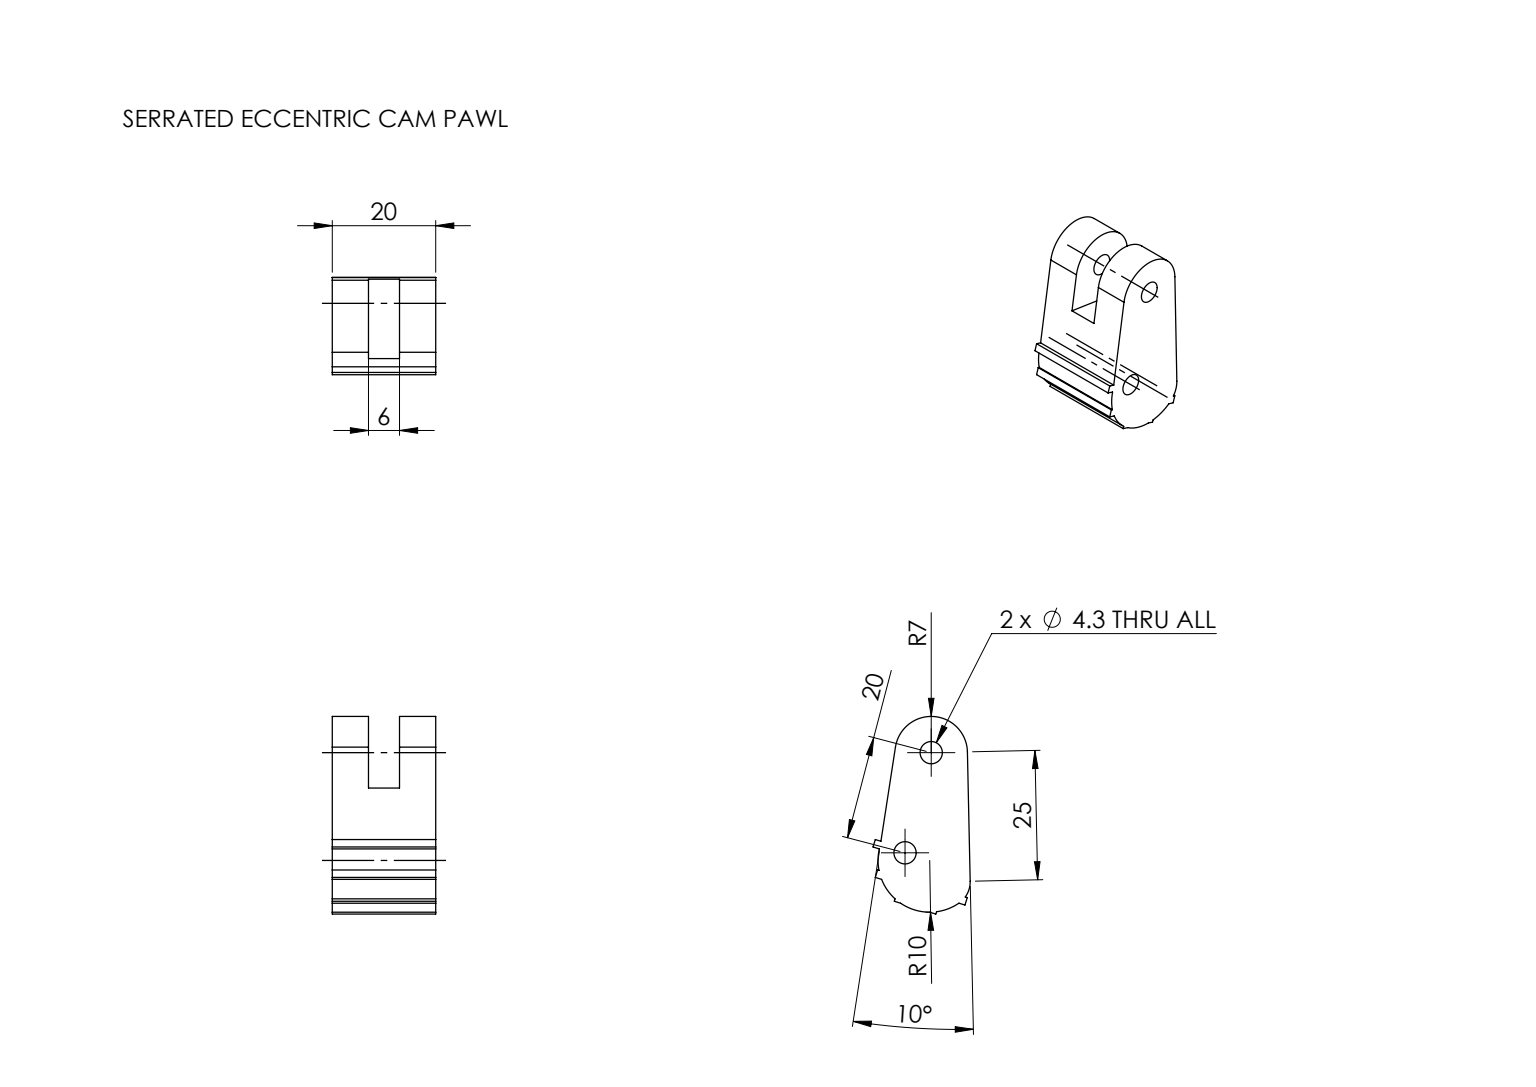
ISO-10303-21;
HEADER;
FILE_DESCRIPTION (('STEP AP214'),
    '1' );
FILE_NAME ('Serrated Eccentric Cam Pawl.step',
    '2026-10-03T20:08:58',
    ( '' ),
    ( '' ),
    'SwSTEP 2.0',
    'SolidWorks 2026',
    '' );
FILE_SCHEMA (( 'AUTOMOTIVE_DESIGN' ));
ENDSEC;

DATA;
#15=PLANE ( 'NONE',  #8371 ) ;
#32=AXIS2_PLACEMENT_3D ( 'NONE', #10637, #3883, #7557 ) ;
#37=ORIENTED_EDGE ( 'NONE', *, *, #5489, .T. ) ;
#60=VECTOR ( 'NONE', #10370, 1000.000000000000000 ) ;
#62=EDGE_CURVE ( 'NONE', #1807, #9471, #2410, .T. ) ;
#89=EDGE_CURVE ( 'NONE', #11132, #9471, #8961, .T. ) ;
#95=CARTESIAN_POINT ( 'NONE',  ( 20.00000000000000000, 39.49790820824818383, -24.06186359251417883 ) ) ;
#99=SHAPE_DEFINITION_REPRESENTATION ( #6268, #1377 ) ;
#101=ORIENTED_EDGE ( 'NONE', *, *, #1479, .F. ) ;
#103=ORIENTED_EDGE ( 'NONE', *, *, #2776, .T. ) ;
#110=ORIENTED_EDGE ( 'NONE', *, *, #895, .F. ) ;
#112=EDGE_CURVE ( 'NONE', #3836, #11042, #11228, .T. ) ;
#118=DIRECTION ( 'NONE',  ( 1.238279320584846685E-16, -0.9554649393887558739, 0.2951046417778634412 ) ) ;
#121=FACE_OUTER_BOUND ( 'NONE', #12151, .T. ) ;
#127=ORIENTED_EDGE ( 'NONE', *, *, #89, .F. ) ;
#135=CARTESIAN_POINT ( 'NONE',  ( 40.00000000000000711, 9.597108420813798446, -18.39576936187866352 ) ) ;
#149=CARTESIAN_POINT ( 'NONE',  ( 20.00000000000000355, 19.99999999999999645, -9.850000000000008527 ) ) ;
#155=ORIENTED_EDGE ( 'NONE', *, *, #11867, .F. ) ;
#170=CARTESIAN_POINT ( 'NONE',  ( 20.00000000000000355, 10.25912655421750230, -11.14847175327133577 ) ) ;
#172=ORIENTED_EDGE ( 'NONE', *, *, #1630, .T. ) ;
#199=AXIS2_PLACEMENT_3D ( 'NONE', #4415, #11118, #3403 ) ;
#205=AXIS2_PLACEMENT_3D ( 'NONE', #5168, #9083, #12128 ) ;
#211=CARTESIAN_POINT ( 'NONE',  ( 27.00000000000000355, 39.34792583643766051, -14.91347054209568945 ) ) ;
#216=CARTESIAN_POINT ( 'NONE',  ( 40.00000000000000000, 39.34792583643765340, -17.06347054209567560 ) ) ;
#220=ADVANCED_FACE ( 'NONE', ( #2602 ), #12455, .T. ) ;
#231=CARTESIAN_POINT ( 'NONE',  ( 40.00000000000000711, 10.63631887905126128, -9.927230231572499619 ) ) ;
#238=ORIENTED_EDGE ( 'NONE', *, *, #6687, .T. ) ;
#243=ORIENTED_EDGE ( 'NONE', *, *, #11135, .T. ) ;
#264=AXIS2_PLACEMENT_3D ( 'NONE', #2269, #10097, #5222 ) ;
#268=EDGE_CURVE ( 'NONE', #6675, #6031, #2672, .T. ) ;
#277=DIRECTION ( 'NONE',  ( -0.000000000000000000, -0.9883022714608525883, 0.1525077710325583313 ) ) ;
#304=EDGE_CURVE ( 'NONE', #11281, #1954, #7365, .T. ) ;
#316=ORIENTED_EDGE ( 'NONE', *, *, #9501, .T. ) ;
#357=LINE ( 'NONE', #2369, #4310 ) ;
#367=ADVANCED_FACE ( 'NONE', ( #4841 ), #6716, .F. ) ;
#385=LINE ( 'NONE', #10217, #5971 ) ;
#407=DIRECTION ( 'NONE',  ( 0.000000000000000000, 1.000000000000000000, 0.000000000000000000 ) ) ;
#416=VECTOR ( 'NONE', #1989, 1000.000000000000114 ) ;
#421=CARTESIAN_POINT ( 'NONE',  ( 40.00000000000000711, 18.52447679111068268, -16.77732469694377926 ) ) ;
#424=ORIENTED_EDGE ( 'NONE', *, *, #89, .T. ) ;
#425=DIRECTION ( 'NONE',  ( 0.000000000000000000, -0.9554649393887557629, 0.2951046417778634412 ) ) ;
#427=ORIENTED_EDGE ( 'NONE', *, *, #12083, .T. ) ;
#430=ORIENTED_EDGE ( 'NONE', *, *, #2792, .F. ) ;
#431=DIRECTION ( 'NONE',  ( 0.000000000000000000, -0.2951046417778627751, -0.9554649393887560960 ) ) ;
#433=SURFACE_SIDE_STYLE ('',( #11389 ) ) ;
#460=VECTOR ( 'NONE', #2524, 1000.000000000000000 ) ;
#463=EDGE_LOOP ( 'NONE', ( #110, #9977 ) ) ;
#484=CYLINDRICAL_SURFACE ( 'NONE', #199, 10.00000000000000000 ) ;
#488=AXIS2_PLACEMENT_3D ( 'NONE', #8589, #5753, #5691 ) ;
#489=FACE_BOUND ( 'NONE', #6630, .T. ) ;
#496=PLANE ( 'NONE',  #10808 ) ;
#500=DIRECTION ( 'NONE',  ( 0.000000000000000000, -0.9554649393887557629, 0.2951046417778634412 ) ) ;
#505=CARTESIAN_POINT ( 'NONE',  ( 20.00000000000000000, 21.12780530657007461, -5.807015647486883481 ) ) ;
#511=CARTESIAN_POINT ( 'NONE',  ( 40.00000000000000711, 15.24625277455639250, -6.248133273622505257 ) ) ;
#553=VECTOR ( 'NONE', #2820, 1000.000000000000114 ) ;
#557=ORIENTED_EDGE ( 'NONE', *, *, #3842, .T. ) ;
#563=VECTOR ( 'NONE', #1495, 1000.000000000000227 ) ;
#567=CARTESIAN_POINT ( 'NONE',  ( 40.00000000000000000, 39.49790820824818383, -24.06186359251417883 ) ) ;
#570=CARTESIAN_POINT ( 'NONE',  ( 40.00000000000000711, 19.99999999999999645, -14.14999999999999147 ) ) ;
#574=VERTEX_POINT ( 'NONE', #5990 ) ;
#575=DIRECTION ( 'NONE',  ( 1.238279320584846685E-16, -0.9554649393887560960, 0.2951046417778627751 ) ) ;
#577=DIRECTION ( 'NONE',  ( -1.000000000000000000, -1.081682119347366197E-16, 6.938893903907228378E-17 ) ) ;
#578=EDGE_CURVE ( 'NONE', #7319, #12298, #9904, .T. ) ;
#580=CYLINDRICAL_SURFACE ( 'NONE', #12033, 2.149999999999992362 ) ;
#614=CARTESIAN_POINT ( 'NONE',  ( 20.00000000000000000, 11.34118543499637077, -24.03007857557328464 ) ) ;
#615=ADVANCED_FACE ( 'NONE', ( #7162 ), #11080, .F. ) ;
#616=CARTESIAN_POINT ( 'NONE',  ( 20.00000000000000355, 18.52447679111067913, -16.77732469694377926 ) ) ;
#621=CIRCLE ( 'NONE', #7816, 9.999999999999998224 ) ;
#642=CARTESIAN_POINT ( 'NONE',  ( 33.00000000000000000, 14.50364731389636397, -24.59751492040896892 ) ) ;
#643=DIRECTION ( 'NONE',  ( 0.000000000000000000, 0.000000000000000000, -1.000000000000000000 ) ) ;
#665=ORIENTED_EDGE ( 'NONE', *, *, #1472, .F. ) ;
#671=CIRCLE ( 'NONE', #10117, 2.149999999999985256 ) ;
#695=EDGE_CURVE ( 'NONE', #11780, #5322, #2587, .T. ) ;
#699=DIRECTION ( 'NONE',  ( 1.000000000000000000, 1.081682119347366197E-16, -6.938893903907228378E-17 ) ) ;
#702=CARTESIAN_POINT ( 'NONE',  ( 27.00000000000000355, 29.58047730022061472, -27.90351864933187898 ) ) ;
#713=CARTESIAN_POINT ( 'NONE',  ( 40.00000000000000711, 11.34118543499637255, -24.03007857557328464 ) ) ;
#725=CARTESIAN_POINT ( 'NONE',  ( 20.00000000000000000, 12.07894703944102766, -21.64141622710139146 ) ) ;
#728=ORIENTED_EDGE ( 'NONE', *, *, #9809, .F. ) ;
#733=LINE ( 'NONE', #12601, #6869 ) ;
#762=CARTESIAN_POINT ( 'NONE',  ( 40.00000000000000711, 10.26855730552414059, -22.42000078613342851 ) ) ;
#767=CARTESIAN_POINT ( 'NONE',  ( 40.00000000000000711, 30.14235464176399404, -24.26236220746664785 ) ) ;
#779=CARTESIAN_POINT ( 'NONE',  ( 20.00000000000000000, 10.63631887905125950, -9.927230231572497843 ) ) ;
#805=CARTESIAN_POINT ( 'NONE',  ( 40.00000000000000711, 11.45997319858344987, -23.64547756539572276 ) ) ;
#821=AXIS2_PLACEMENT_3D ( 'NONE', #5989, #11671, #5736 ) ;
#824=EDGE_CURVE ( 'NONE', #7005, #11281, #3866, .T. ) ;
#850=DIRECTION ( 'NONE',  ( 1.000000000000000000, -0.000000000000000000, -6.938893903907228378E-17 ) ) ;
#862=ORIENTED_EDGE ( 'NONE', *, *, #6687, .F. ) ;
#872=EDGE_CURVE ( 'NONE', #5322, #574, #6832, .T. ) ;
#876=LINE ( 'NONE', #4088, #7398 ) ;
#879=EDGE_LOOP ( 'NONE', ( #430, #5834, #11812, #1139 ) ) ;
#895=EDGE_CURVE ( 'NONE', #6619, #5731, #4929, .T. ) ;
#913=VECTOR ( 'NONE', #8680, 1000.000000000000000 ) ;
#915=DIRECTION ( 'NONE',  ( -1.000000000000000000, -1.081682119347366197E-16, 6.938893903907228378E-17 ) ) ;
#923=CARTESIAN_POINT ( 'NONE',  ( 20.00000000000000000, 8.163911011730665024, -17.95311239921186441 ) ) ;
#925=EDGE_CURVE ( 'NONE', #10658, #2655, #357, .T. ) ;
#938=VERTEX_POINT ( 'NONE', #7194 ) ;
#946=DIRECTION ( 'NONE',  ( -1.081682119347366197E-16, 1.000000000000000000, 0.000000000000000000 ) ) ;
#948=ADVANCED_FACE ( 'NONE', ( #3466 ), #484, .T. ) ;
#950=ORIENTED_EDGE ( 'NONE', *, *, #1873, .F. ) ;
#964=EDGE_CURVE ( 'NONE', #11709, #1279, #2236, .T. ) ;
#970=DIRECTION ( 'NONE',  ( 7.169062767534772867E-17, -0.02142605311579142552, 0.9997704357740727632 ) ) ;
#997=EDGE_CURVE ( 'NONE', #3286, #9151, #3483, .T. ) ;
#1008=EDGE_LOOP ( 'NONE', ( #5764, #10223, #12292, #11299 ) ) ;
#1031=CARTESIAN_POINT ( 'NONE',  ( 40.00000000000000711, 14.50364731389636574, -24.59751492040896892 ) ) ;
#1037=CYLINDRICAL_SURFACE ( 'NONE', #1434, 10.00000000000000000 ) ;
#1101=DIRECTION ( 'NONE',  ( 1.238279320584846685E-16, -0.9554649393887560960, 0.2951046417778627751 ) ) ;
#1122=ORIENTED_EDGE ( 'NONE', *, *, #9718, .T. ) ;
#1131=CARTESIAN_POINT ( 'NONE',  ( 20.00000000000000355, 19.99999999999999645, -12.00000000000000000 ) ) ;
#1138=VECTOR ( 'NONE', #1770, 1000.000000000000000 ) ;
#1139=ORIENTED_EDGE ( 'NONE', *, *, #8439, .F. ) ;
#1152=CARTESIAN_POINT ( 'NONE',  ( 40.00000000000000711, 8.524476791110680907, -16.77732469694377926 ) ) ;
#1163=CARTESIAN_POINT ( 'NONE',  ( 20.00000000000000000, 15.24625277455639072, -6.248133273622503481 ) ) ;
#1190=DIRECTION ( 'NONE',  ( 1.000000000000000000, -0.000000000000000000, -6.938893903907228378E-17 ) ) ;
#1192=DIRECTION ( 'NONE',  ( 1.000000000000000000, 1.081682119347366197E-16, -6.938893903907228378E-17 ) ) ;
#1195=EDGE_CURVE ( 'NONE', #8729, #11132, #8527, .T. ) ;
#1202=DIRECTION ( 'NONE',  ( 0.000000000000000000, 1.000000000000000000, 0.000000000000000000 ) ) ;
#1205=CIRCLE ( 'NONE', #11288, 9.999999999999998224 ) ;
#1212=CIRCLE ( 'NONE', #9019, 2.149999999999985256 ) ;
#1235=EDGE_LOOP ( 'NONE', ( #8347, #1122, #10045, #7560 ) ) ;
#1245=EDGE_CURVE ( 'NONE', #6857, #5859, #1205, .T. ) ;
#1251=CARTESIAN_POINT ( 'NONE',  ( 40.00000000000000000, 39.34792583643766051, -14.91347054209569301 ) ) ;
#1254=ORIENTED_EDGE ( 'NONE', *, *, #1536, .F. ) ;
#1258=DIRECTION ( 'NONE',  ( 1.000000000000000000, 1.081682119347366321E-16, -6.938893903907228378E-17 ) ) ;
#1279=VERTEX_POINT ( 'NONE', #1952 ) ;
#1322=CARTESIAN_POINT ( 'NONE',  ( 40.00000000000000000, 39.34792583643766051, -19.21347054209566352 ) ) ;
#1323=DIRECTION ( 'NONE',  ( -3.437775699846489820E-17, -0.2951046417778627751, -0.9554649393887560960 ) ) ;
#1333=LINE ( 'NONE', #5084, #4298 ) ;
#1340=CYLINDRICAL_SURFACE ( 'NONE', #12047, 10.00000000000000000 ) ;
#1348=CARTESIAN_POINT ( 'NONE',  ( 40.00000000000000711, 10.63631887905126128, -9.927230231572499619 ) ) ;
#1377=SHAPE_REPRESENTATION ( 'Serrated Eccentric Cam Pawl', ( #12422 ), #2062 ) ;
#1394=EDGE_CURVE ( 'NONE', #8136, #2021, #2508, .T. ) ;
#1410=DIRECTION ( 'NONE',  ( 1.000000000000000000, 1.081682119347366321E-16, -6.938893903907228378E-17 ) ) ;
#1427=VERTEX_POINT ( 'NONE', #7520 ) ;
#1434=AXIS2_PLACEMENT_3D ( 'NONE', #9786, #915, #4065 ) ;
#1438=ORIENTED_EDGE ( 'NONE', *, *, #11480, .F. ) ;
#1442=MECHANICAL_DESIGN_GEOMETRIC_PRESENTATION_REPRESENTATION('',(#12570),#6396);
#1462=LINE ( 'NONE', #3417, #2826 ) ;
#1472=EDGE_CURVE ( 'NONE', #11132, #938, #6627, .T. ) ;
#1479=EDGE_CURVE ( 'NONE', #6979, #2021, #10668, .T. ) ;
#1495=DIRECTION ( 'NONE',  ( 2.187388225841179596E-16, -0.9997704357740726522, -0.02142605311579142552 ) ) ;
#1499=CARTESIAN_POINT ( 'NONE',  ( 20.00000000000000000, 21.12780530657007461, -5.807015647486883481 ) ) ;
#1517=EDGE_LOOP ( 'NONE', ( #10586, #238, #7027, #9677, #2521, #5666, #4792, #7574 ) ) ;
#1536=EDGE_CURVE ( 'NONE', #4933, #5862, #5134, .T. ) ;
#1546=VECTOR ( 'NONE', #10772, 1000.000000000000000 ) ;
#1555=DIRECTION ( 'NONE',  ( 1.000000000000000000, 1.081682119347366197E-16, -6.938893903907228378E-17 ) ) ;
#1560=CARTESIAN_POINT ( 'NONE',  ( 20.00000000000000355, 8.611173066148735344, -18.09125363591105540 ) ) ;
#1563=CYLINDRICAL_SURFACE ( 'NONE', #12684, 5.000000000000000888 ) ;
#1589=DIRECTION ( 'NONE',  ( -1.081682119347366197E-16, 1.000000000000000000, 0.000000000000000000 ) ) ;
#1597=VECTOR ( 'NONE', #10603, 1000.000000000000000 ) ;
#1599=CARTESIAN_POINT ( 'NONE',  ( 40.00000000000000711, 22.22477142302764364, -7.338293953734280173 ) ) ;
#1630=EDGE_CURVE ( 'NONE', #6277, #6857, #876, .T. ) ;
#1651=AXIS2_PLACEMENT_3D ( 'NONE', #11186, #8281, #2434 ) ;
#1656=DIRECTION ( 'NONE',  ( 1.000000000000000000, 1.081682119347366197E-16, -6.938893903907228378E-17 ) ) ;
#1698=EDGE_LOOP ( 'NONE', ( #12167, #10076, #4423, #3828 ) ) ;
#1714=ORIENTED_EDGE ( 'NONE', *, *, #8066, .F. ) ;
#1715=ORIENTED_EDGE ( 'NONE', *, *, #3433, .F. ) ;
#1735=CARTESIAN_POINT ( 'NONE',  ( 40.00000000000000711, 12.07894703944102943, -21.64141622710139146 ) ) ;
#1737=DIRECTION ( 'NONE',  ( 0.000000000000000000, 0.000000000000000000, -1.000000000000000000 ) ) ;
#1770=DIRECTION ( 'NONE',  ( 1.238279320584846685E-16, -0.9554649393887558739, 0.2951046417778634412 ) ) ;
#1772=STYLED_ITEM ( 'NONE', ( #12365 ), #5705 ) ;
#1776=CARTESIAN_POINT ( 'NONE',  ( 20.00000000000000000, 10.63631887905125950, -9.927230231572497843 ) ) ;
#1799=CARTESIAN_POINT ( 'NONE',  ( 20.00000000000000000, 10.64574963035789601, -21.19875926443459591 ) ) ;
#1807=VERTEX_POINT ( 'NONE', #12615 ) ;
#1819=FACE_OUTER_BOUND ( 'NONE', #3970, .T. ) ;
#1822=VERTEX_POINT ( 'NONE', #10654 ) ;
#1839=EDGE_CURVE ( 'NONE', #5204, #2655, #5643, .T. ) ;
#1869=CARTESIAN_POINT ( 'NONE',  ( 40.00000000000000711, 14.86906044972264240, -7.469374795321334304 ) ) ;
#1873=EDGE_CURVE ( 'NONE', #9471, #9760, #10978, .T. ) ;
#1899=ORIENTED_EDGE ( 'NONE', *, *, #578, .T. ) ;
#1915=ORIENTED_EDGE ( 'NONE', *, *, #2093, .T. ) ;
#1952=CARTESIAN_POINT ( 'NONE',  ( 40.00000000000000711, 10.25912655421750230, -11.14847175327134110 ) ) ;
#1954=VERTEX_POINT ( 'NONE', #11894 ) ;
#1984=CIRCLE ( 'NONE', #6311, 2.149999999999985256 ) ;
#1986=CARTESIAN_POINT ( 'NONE',  ( 32.99999999999999289, 39.34792583643766051, -14.91347054209568945 ) ) ;
#1989=DIRECTION ( 'NONE',  ( -0.000000000000000000, -0.9883022714608525883, 0.1525077710325583313 ) ) ;
#1993=EDGE_LOOP ( 'NONE', ( #10669, #10613, #8744, #5830 ) ) ;
#2003=DIRECTION ( 'NONE',  ( -3.437775699846489820E-17, -0.2951046417778627751, -0.9554649393887560960 ) ) ;
#2004=PLANE ( 'NONE',  #7497 ) ;
#2021=VERTEX_POINT ( 'NONE', #1251 ) ;
#2023=ORIENTED_EDGE ( 'NONE', *, *, #11135, .F. ) ;
#2026=DIRECTION ( 'NONE',  ( -3.437775699846489820E-17, -0.2951046417778627751, -0.9554649393887560960 ) ) ;
#2047=VECTOR ( 'NONE', #3153, 1000.000000000000114 ) ;
#2049=CARTESIAN_POINT ( 'NONE',  ( 20.00000000000000000, 11.10553687445042570, -10.07215277424222855 ) ) ;
#2062=( GEOMETRIC_REPRESENTATION_CONTEXT ( 3 ) GLOBAL_UNCERTAINTY_ASSIGNED_CONTEXT ( ( #5469 ) ) GLOBAL_UNIT_ASSIGNED_CONTEXT ( ( #2406, #6390, #11551 ) ) REPRESENTATION_CONTEXT ( 'NONE', 'WORKASPACE' ) );
#2075=CARTESIAN_POINT ( 'NONE',  ( 20.00000000000000000, 15.24625277455639072, -6.248133273622503481 ) ) ;
#2093=EDGE_CURVE ( 'NONE', #6823, #9939, #4104, .T. ) ;
#2103=LINE ( 'NONE', #4160, #8896 ) ;
#2127=VERTEX_POINT ( 'NONE', #6657 ) ;
#2147=EDGE_CURVE ( 'NONE', #12369, #1954, #4712, .T. ) ;
#2148=DIRECTION ( 'NONE',  ( -1.000000000000000000, -2.206481006425900381E-16, 8.674603474570137221E-17 ) ) ;
#2153=EDGE_LOOP ( 'NONE', ( #101, #3167 ) ) ;
#2165=CARTESIAN_POINT ( 'NONE',  ( 40.00000000000000711, 22.56100271565320980, -6.249672610153679919 ) ) ;
#2181=CARTESIAN_POINT ( 'NONE',  ( 27.00000000000000355, 39.34792583643766051, -17.06347054209567915 ) ) ;
#2190=FACE_OUTER_BOUND ( 'NONE', #11323, .T. ) ;
#2193=ADVANCED_FACE ( 'NONE', ( #3115 ), #11861, .T. ) ;
#2206=ADVANCED_BREP_SHAPE_REPRESENTATION ( '', ( #5705, #12422 ), #2062 ) ;
#2209=CARTESIAN_POINT ( 'NONE',  ( 32.99999999999999289, 39.34792583643766051, -19.21347054209566707 ) ) ;
#2225=DIRECTION ( 'NONE',  ( 0.000000000000000000, -1.000000000000000000, 0.000000000000000000 ) ) ;
#2226=ORIENTED_EDGE ( 'NONE', *, *, #7584, .T. ) ;
#2232=EDGE_LOOP ( 'NONE', ( #3487, #155, #2650, #1915 ) ) ;
#2236=LINE ( 'NONE', #231, #4108 ) ;
#2246=CARTESIAN_POINT ( 'NONE',  ( 40.00000000000000711, 14.86906044972263707, -7.469374795321336080 ) ) ;
#2269=CARTESIAN_POINT ( 'NONE',  ( 40.00000000000000000, 39.34792583643766051, -17.06347054209567915 ) ) ;
#2289=DIRECTION ( 'NONE',  ( -1.000000000000000000, -1.081682119347366197E-16, 6.938893903907228378E-17 ) ) ;
#2308=ORIENTED_EDGE ( 'NONE', *, *, #9718, .F. ) ;
#2323=FACE_OUTER_BOUND ( 'NONE', #2841, .T. ) ;
#2329=DIRECTION ( 'NONE',  ( -3.437775699846489820E-17, -0.2951046417778627751, -0.9554649393887560960 ) ) ;
#2369=CARTESIAN_POINT ( 'NONE',  ( 20.00000000000000000, 10.63631887905125950, -9.927230231572497843 ) ) ;
#2370=FACE_OUTER_BOUND ( 'NONE', #9107, .T. ) ;
#2373=PLANE ( 'NONE',  #10491 ) ;
#2401=FACE_OUTER_BOUND ( 'NONE', #9363, .T. ) ;
#2406=( LENGTH_UNIT ( ) NAMED_UNIT ( * ) SI_UNIT ( .MILLI., .METRE. ) );
#2410=LINE ( 'NONE', #11095, #4379 ) ;
#2420=FACE_OUTER_BOUND ( 'NONE', #6608, .T. ) ;
#2428=CARTESIAN_POINT ( 'NONE',  ( 20.00000000000000355, 19.99999999999999645, -12.00000000000000000 ) ) ;
#2432=EDGE_CURVE ( 'NONE', #8348, #4291, #385, .T. ) ;
#2434=DIRECTION ( 'NONE',  ( 0.000000000000000000, -1.000000000000000000, 0.000000000000000000 ) ) ;
#2439=EDGE_CURVE ( 'NONE', #8682, #11780, #6642, .T. ) ;
#2451=VERTEX_POINT ( 'NONE', #4642 ) ;
#2480=EDGE_CURVE ( 'NONE', #3728, #7005, #3105, .T. ) ;
#2483=CARTESIAN_POINT ( 'NONE',  ( 40.00000000000000000, 39.49790820824818383, -24.06186359251417883 ) ) ;
#2504=ORIENTED_EDGE ( 'NONE', *, *, #6586, .T. ) ;
#2506=FACE_BOUND ( 'NONE', #463, .T. ) ;
#2508=LINE ( 'NONE', #2712, #7385 ) ;
#2520=EDGE_CURVE ( 'NONE', #574, #12468, #4580, .T. ) ;
#2521=ORIENTED_EDGE ( 'NONE', *, *, #5672, .F. ) ;
#2524=DIRECTION ( 'NONE',  ( -1.238279320584846685E-16, 0.9554649393887558739, -0.2951046417778634412 ) ) ;
#2550=EDGE_CURVE ( 'NONE', #11042, #11825, #10490, .T. ) ;
#2554=CARTESIAN_POINT ( 'NONE',  ( 20.00000000000000000, 16.59466514679920124, -6.965300083364789785 ) ) ;
#2562=ORIENTED_EDGE ( 'NONE', *, *, #5672, .T. ) ;
#2587=LINE ( 'NONE', #642, #11771 ) ;
#2602=FACE_OUTER_BOUND ( 'NONE', #12626, .T. ) ;
#2603=COLOUR_RGB ( '', 0.31764706, 0.68627451, 0.89019608) ;
#2604=CARTESIAN_POINT ( 'NONE',  ( 20.00000000000000355, 11.45997319858344810, -23.64547756539571566 ) ) ;
#2610=VECTOR ( 'NONE', #10522, 1000.000000000000000 ) ;
#2624=EDGE_CURVE ( 'NONE', #8729, #1807, #5914, .T. ) ;
#2629=CARTESIAN_POINT ( 'NONE',  ( 40.00000000000000711, 21.12780530657007816, -5.807015647486885257 ) ) ;
#2637=EDGE_CURVE ( 'NONE', #2127, #6031, #2789, .T. ) ;
#2644=EDGE_CURVE ( 'NONE', #1822, #11190, #12694, .T. ) ;
#2650=ORIENTED_EDGE ( 'NONE', *, *, #7602, .T. ) ;
#2655=VERTEX_POINT ( 'NONE', #2049 ) ;
#2665=PRESENTATION_STYLE_ASSIGNMENT (( #9584 ) ) ;
#2671=VECTOR ( 'NONE', #10863, 1000.000000000000000 ) ;
#2672=LINE ( 'NONE', #6394, #4168 ) ;
#2673=CARTESIAN_POINT ( 'NONE',  ( 40.00000000000000711, 19.99999999999999645, -12.00000000000000178 ) ) ;
#2689=ORIENTED_EDGE ( 'NONE', *, *, #4520, .T. ) ;
#2700=ORIENTED_EDGE ( 'NONE', *, *, #7431, .T. ) ;
#2712=CARTESIAN_POINT ( 'NONE',  ( 40.00000000000000000, 39.34792583643766051, -14.91347054209568945 ) ) ;
#2727=ADVANCED_FACE ( 'NONE', ( #3355 ), #3168, .F. ) ;
#2732=ORIENTED_EDGE ( 'NONE', *, *, #3539, .F. ) ;
#2768=ORIENTED_EDGE ( 'NONE', *, *, #9825, .T. ) ;
#2769=DIRECTION ( 'NONE',  ( -3.437775699846481192E-17, -0.2951046417778634967, -0.9554649393887558739 ) ) ;
#2776=EDGE_CURVE ( 'NONE', #11825, #1954, #1333, .T. ) ;
#2789=LINE ( 'NONE', #4767, #2671 ) ;
#2792=EDGE_CURVE ( 'NONE', #10595, #4775, #12045, .T. ) ;
#2800=CARTESIAN_POINT ( 'NONE',  ( 40.00000000000000711, 10.64574963035789779, -21.19875926443459591 ) ) ;
#2804=VECTOR ( 'NONE', #12374, 1000.000000000000114 ) ;
#2807=AXIS2_PLACEMENT_3D ( 'NONE', #6219, #3406, #425 ) ;
#2820=DIRECTION ( 'NONE',  ( -3.437775699846489820E-17, -0.2951046417778627751, -0.9554649393887560960 ) ) ;
#2826=VECTOR ( 'NONE', #7333, 1000.000000000000000 ) ;
#2841=EDGE_LOOP ( 'NONE', ( #12665, #10276, #10719, #8806 ) ) ;
#2852=ORIENTED_EDGE ( 'NONE', *, *, #5325, .F. ) ;
#2854=ORIENTED_EDGE ( 'NONE', *, *, #10288, .F. ) ;
#2873=UNCERTAINTY_MEASURE_WITH_UNIT (LENGTH_MEASURE( 1.000000000000000082E-05 ), #11195, 'distance_accuracy_value', 'NONE');
#2898=DIRECTION ( 'NONE',  ( -1.000000000000000000, -1.081682119347366197E-16, 6.938893903907228378E-17 ) ) ;
#2899=ORIENTED_EDGE ( 'NONE', *, *, #6245, .T. ) ;
#2911=ORIENTED_EDGE ( 'NONE', *, *, #10731, .T. ) ;
#2919=EDGE_CURVE ( 'NONE', #6872, #11175, #6360, .T. ) ;
#2936=DIRECTION ( 'NONE',  ( -1.000000000000000000, -2.206481006425900381E-16, 8.674603474570138454E-17 ) ) ;
#2938=AXIS2_PLACEMENT_3D ( 'NONE', #1031, #970, #8643 ) ;
#2951=DIRECTION ( 'NONE',  ( 0.000000000000000000, -0.2951046417778627751, -0.9554649393887560960 ) ) ;
#2956=ORIENTED_EDGE ( 'NONE', *, *, #2432, .T. ) ;
#3016=ORIENTED_EDGE ( 'NONE', *, *, #925, .F. ) ;
#3024=DIRECTION ( 'NONE',  ( -1.000000000000000000, -1.081682119347366197E-16, 6.938893903907228378E-17 ) ) ;
#3028=CARTESIAN_POINT ( 'NONE',  ( 40.00000000000000711, 19.99999999999999645, -9.850000000000010303 ) ) ;
#3038=DIRECTION ( 'NONE',  ( 1.000000000000000000, 1.081682119347366321E-16, -6.938893903907228378E-17 ) ) ;
#3087=AXIS2_PLACEMENT_3D ( 'NONE', #11131, #4300, #8164 ) ;
#3088=CARTESIAN_POINT ( 'NONE',  ( 40.00000000000000000, 39.34792583643766051, -17.06347054209567915 ) ) ;
#3105=CIRCLE ( 'NONE', #4536, 9.999999999999998224 ) ;
#3115=FACE_OUTER_BOUND ( 'NONE', #879, .T. ) ;
#3139=DIRECTION ( 'NONE',  ( 1.238279320584846685E-16, -0.9554649393887560960, 0.2951046417778627751 ) ) ;
#3153=DIRECTION ( 'NONE',  ( -3.437775699846489820E-17, -0.2951046417778627751, -0.9554649393887560960 ) ) ;
#3162=ORIENTED_EDGE ( 'NONE', *, *, #1839, .T. ) ;
#3167=ORIENTED_EDGE ( 'NONE', *, *, #12083, .F. ) ;
#3168=PLANE ( 'NONE',  #3087 ) ;
#3195=FACE_BOUND ( 'NONE', #9629, .T. ) ;
#3203=EDGE_CURVE ( 'NONE', #9222, #6979, #2103, .T. ) ;
#3205=CARTESIAN_POINT ( 'NONE',  ( 40.00000000000000711, 14.39651704831740986, -19.59866274153860388 ) ) ;
#3209=ORIENTED_EDGE ( 'NONE', *, *, #2644, .T. ) ;
#3221=LINE ( 'NONE', #9941, #7769 ) ;
#3225=CIRCLE ( 'NONE', #10383, 2.149999999999988809 ) ;
#3241=CARTESIAN_POINT ( 'NONE',  ( 20.00000000000000000, 9.597108420813796670, -18.39576936187866352 ) ) ;
#3258=EDGE_CURVE ( 'NONE', #9939, #10595, #12628, .T. ) ;
#3272=ORIENTED_EDGE ( 'NONE', *, *, #62, .T. ) ;
#3286=VERTEX_POINT ( 'NONE', #9409 ) ;
#3288=LINE ( 'NONE', #9182, #11387 ) ;
#3297=CARTESIAN_POINT ( 'NONE',  ( 20.00000000000000355, 14.50364731389636397, -24.59751492040896892 ) ) ;
#3329=CARTESIAN_POINT ( 'NONE',  ( 40.00000000000000711, 21.47552320888931021, -7.222675303056226070 ) ) ;
#3344=CARTESIAN_POINT ( 'NONE',  ( 20.00000000000000000, 10.63631887905125950, -9.927230231572497843 ) ) ;
#3355=FACE_OUTER_BOUND ( 'NONE', #3473, .T. ) ;
#3403=DIRECTION ( 'NONE',  ( 0.000000000000000000, -1.000000000000000000, 0.000000000000000000 ) ) ;
#3406=DIRECTION ( 'NONE',  ( 3.437775699846481192E-17, 0.2951046417778634967, 0.9554649393887558739 ) ) ;
#3415=DIRECTION ( 'NONE',  ( -1.000000000000000000, -2.206481006425900381E-16, 8.674603474570138454E-17 ) ) ;
#3417=CARTESIAN_POINT ( 'NONE',  ( 40.00000000000000711, 22.22477142302764008, -7.338293953734282837 ) ) ;
#3433=EDGE_CURVE ( 'NONE', #5862, #6619, #733, .T. ) ;
#3436=VECTOR ( 'NONE', #4384, 1000.000000000000000 ) ;
#3441=CARTESIAN_POINT ( 'NONE',  ( 40.00000000000000711, 8.611173066148737121, -18.09125363591105540 ) ) ;
#3450=FACE_OUTER_BOUND ( 'NONE', #12688, .T. ) ;
#3454=DIRECTION ( 'NONE',  ( 1.238279320584846685E-16, -0.9554649393887560960, 0.2951046417778627751 ) ) ;
#3466=FACE_OUTER_BOUND ( 'NONE', #4679, .T. ) ;
#3473=EDGE_LOOP ( 'NONE', ( #6548, #2562, #665, #424 ) ) ;
#3481=FACE_OUTER_BOUND ( 'NONE', #1993, .T. ) ;
#3483=CIRCLE ( 'NONE', #6962, 2.149999999999985256 ) ;
#3485=DIRECTION ( 'NONE',  ( 0.000000000000000000, -1.000000000000000000, 0.000000000000000000 ) ) ;
#3487=ORIENTED_EDGE ( 'NONE', *, *, #12307, .F. ) ;
#3489=DIRECTION ( 'NONE',  ( 0.000000000000000000, 1.000000000000000000, 0.000000000000000000 ) ) ;
#3498=PLANE ( 'NONE',  #205 ) ;
#3500=VECTOR ( 'NONE', #11205, 1000.000000000000000 ) ;
#3539=EDGE_CURVE ( 'NONE', #11717, #12369, #12634, .T. ) ;
#3568=DIRECTION ( 'NONE',  ( -1.000000000000000000, -1.081682119347366197E-16, 6.938893903907228378E-17 ) ) ;
#3599=FILL_AREA_STYLE_COLOUR ( '', #2603 ) ;
#3600=ORIENTED_EDGE ( 'NONE', *, *, #12188, .T. ) ;
#3609=DIRECTION ( 'NONE',  ( -3.437775699846489820E-17, -0.2951046417778627751, -0.9554649393887560960 ) ) ;
#3614=CARTESIAN_POINT ( 'NONE',  ( 20.00000000000000000, 39.34792583643765340, -17.06347054209567560 ) ) ;
#3620=ADVANCED_FACE ( 'NONE', ( #3195, #11942 ), #4204, .T. ) ;
#3635=DIRECTION ( 'NONE',  ( -1.000000000000000000, -1.081682119347366197E-16, 6.938893903907228378E-17 ) ) ;
#3646=DIRECTION ( 'NONE',  ( 1.238279320584846685E-16, -0.9554649393887560960, 0.2951046417778627751 ) ) ;
#3647=CARTESIAN_POINT ( 'NONE',  ( 20.00000000000000000, 21.12780530657007461, -5.807015647486883481 ) ) ;
#3668=CARTESIAN_POINT ( 'NONE',  ( 40.00000000000000711, 32.50906206197875292, -8.925292473609246713 ) ) ;
#3691=CARTESIAN_POINT ( 'NONE',  ( 20.00000000000000000, 9.907988025913237351, -23.58742161290648554 ) ) ;
#3704=VECTOR ( 'NONE', #11968, 1000.000000000000000 ) ;
#3722=VECTOR ( 'NONE', #8494, 1000.000000000000114 ) ;
#3728=VERTEX_POINT ( 'NONE', #1560 ) ;
#3745=VECTOR ( 'NONE', #3762, 1000.000000000000000 ) ;
#3762=DIRECTION ( 'NONE',  ( -1.238279320584846685E-16, 0.9554649393887558739, -0.2951046417778634412 ) ) ;
#3772=ORIENTED_EDGE ( 'NONE', *, *, #1394, .T. ) ;
#3790=LINE ( 'NONE', #3668, #913 ) ;
#3798=ORIENTED_EDGE ( 'NONE', *, *, #112, .F. ) ;
#3799=DIRECTION ( 'NONE',  ( 1.000000000000000000, 1.081682119347366321E-16, -6.938893903907228378E-17 ) ) ;
#3813=FILL_AREA_STYLE_COLOUR ( '', #5353 ) ;
#3821=FACE_OUTER_BOUND ( 'NONE', #11173, .T. ) ;
#3822=DIRECTION ( 'NONE',  ( 0.000000000000000000, -1.000000000000000000, 0.000000000000000000 ) ) ;
#3828=ORIENTED_EDGE ( 'NONE', *, *, #8453, .T. ) ;
#3836=VERTEX_POINT ( 'NONE', #2604 ) ;
#3842=EDGE_CURVE ( 'NONE', #12369, #7005, #4530, .T. ) ;
#3844=EDGE_CURVE ( 'NONE', #8348, #5859, #7487, .T. ) ;
#3858=ORIENTED_EDGE ( 'NONE', *, *, #7814, .F. ) ;
#3866=LINE ( 'NONE', #1799, #2047 ) ;
#3871=LINE ( 'NONE', #4899, #416 ) ;
#3882=PLANE ( 'NONE',  #8832 ) ;
#3883=DIRECTION ( 'NONE',  ( -3.437775699846481192E-17, -0.2951046417778634967, -0.9554649393887558739 ) ) ;
#3919=EDGE_LOOP ( 'NONE', ( #5532, #7042, #12541, #10161 ) ) ;
#3922=ADVANCED_FACE ( 'NONE', ( #121 ), #11673, .F. ) ;
#3947=CIRCLE ( 'NONE', #10935, 10.00000000000000178 ) ;
#3959=PLANE ( 'NONE',  #9456 ) ;
#3967=EDGE_CURVE ( 'NONE', #10658, #11709, #12518, .T. ) ;
#3970=EDGE_LOOP ( 'NONE', ( #3272, #127, #9553, #10244 ) ) ;
#3992=ORIENTED_EDGE ( 'NONE', *, *, #2480, .F. ) ;
#4019=CARTESIAN_POINT ( 'NONE',  ( 20.00000000000000000, 12.07894703944102766, -21.64141622710139146 ) ) ;
#4052=ORIENTED_EDGE ( 'NONE', *, *, #2147, .F. ) ;
#4065=DIRECTION ( 'NONE',  ( 0.000000000000000000, -1.000000000000000000, 0.000000000000000000 ) ) ;
#4075=EDGE_LOOP ( 'NONE', ( #7755, #12731 ) ) ;
#4081=ORIENTED_EDGE ( 'NONE', *, *, #11867, .T. ) ;
#4088=CARTESIAN_POINT ( 'NONE',  ( 40.00000000000000711, 20.75061298173632451, -7.028257169185713416 ) ) ;
#4095=CARTESIAN_POINT ( 'NONE',  ( 27.00000000000000355, 39.49790820824818383, -24.06186359251417883 ) ) ;
#4103=VECTOR ( 'NONE', #4661, 1000.000000000000114 ) ;
#4104=CIRCLE ( 'NONE', #5338, 9.999999999999998224 ) ;
#4108=VECTOR ( 'NONE', #6282, 1000.000000000000114 ) ;
#4113=VECTOR ( 'NONE', #1323, 1000.000000000000114 ) ;
#4120=ORIENTED_EDGE ( 'NONE', *, *, #8066, .T. ) ;
#4130=CARTESIAN_POINT ( 'NONE',  ( 40.00000000000000711, 16.59466514679920479, -6.965300083364795114 ) ) ;
#4133=CARTESIAN_POINT ( 'NONE',  ( 40.00000000000000000, 39.34792583643766051, -17.06347054209567915 ) ) ;
#4160=CARTESIAN_POINT ( 'NONE',  ( 40.00000000000000000, 39.34792583643766051, -19.21347054209566707 ) ) ;
#4163=CARTESIAN_POINT ( 'NONE',  ( 20.00000000000000000, 39.34792583643766051, -17.06347054209567915 ) ) ;
#4168=VECTOR ( 'NONE', #10503, 1000.000000000000000 ) ;
#4204=PLANE ( 'NONE',  #7882 ) ;
#4212=FACE_OUTER_BOUND ( 'NONE', #4560, .T. ) ;
#4224=DIRECTION ( 'NONE',  ( 0.000000000000000000, 1.000000000000000000, 0.000000000000000000 ) ) ;
#4227=LINE ( 'NONE', #8151, #9755 ) ;
#4265=CARTESIAN_POINT ( 'NONE',  ( 40.00000000000000711, 11.45997319858345342, -23.64547756539571566 ) ) ;
#4281=ADVANCED_FACE ( 'NONE', ( #3481 ), #4690, .F. ) ;
#4291=VERTEX_POINT ( 'NONE', #4815 ) ;
#4298=VECTOR ( 'NONE', #118, 1000.000000000000000 ) ;
#4300=DIRECTION ( 'NONE',  ( 1.238279320584846685E-16, -0.9554649393887560960, 0.2951046417778627751 ) ) ;
#4310=VECTOR ( 'NONE', #12221, 1000.000000000000000 ) ;
#4317=EDGE_CURVE ( 'NONE', #4933, #5731, #10790, .T. ) ;
#4330=DIRECTION ( 'NONE',  ( 1.000000000000000000, 1.081682119347366197E-16, -6.938893903907228378E-17 ) ) ;
#4348=CARTESIAN_POINT ( 'NONE',  ( 20.00000000000000355, 18.52447679111067913, -16.77732469694377926 ) ) ;
#4351=EDGE_CURVE ( 'NONE', #5322, #2127, #5773, .T. ) ;
#4379=VECTOR ( 'NONE', #5234, 1000.000000000000000 ) ;
#4384=DIRECTION ( 'NONE',  ( -1.238279320584846685E-16, 0.9554649393887558739, -0.2951046417778634412 ) ) ;
#4388=ORIENTED_EDGE ( 'NONE', *, *, #4600, .F. ) ;
#4403=CARTESIAN_POINT ( 'NONE',  ( 20.00000000000000000, 10.64574963035789601, -21.19875926443459591 ) ) ;
#4414=DIRECTION ( 'NONE',  ( 1.000000000000000000, 1.081682119347366197E-16, -6.938893903907228378E-17 ) ) ;
#4415=CARTESIAN_POINT ( 'NONE',  ( 40.00000000000000711, 18.52447679111068268, -16.77732469694377926 ) ) ;
#4419=FACE_OUTER_BOUND ( 'NONE', #9756, .T. ) ;
#4420=ORIENTED_EDGE ( 'NONE', *, *, #2432, .F. ) ;
#4423=ORIENTED_EDGE ( 'NONE', *, *, #2624, .F. ) ;
#4425=ORIENTED_EDGE ( 'NONE', *, *, #2439, .F. ) ;
#4441=ORIENTED_EDGE ( 'NONE', *, *, #7038, .T. ) ;
#4444=FACE_OUTER_BOUND ( 'NONE', #8973, .T. ) ;
#4466=DIRECTION ( 'NONE',  ( 1.000000000000000000, -0.000000000000000000, -6.938893903907228378E-17 ) ) ;
#4494=CARTESIAN_POINT ( 'NONE',  ( 40.00000000000000000, 39.34792583643766051, -17.06347054209567915 ) ) ;
#4495=FACE_OUTER_BOUND ( 'NONE', #12217, .T. ) ;
#4496=ORIENTED_EDGE ( 'NONE', *, *, #1394, .F. ) ;
#4515=CARTESIAN_POINT ( 'NONE',  ( 40.00000000000000711, 19.99999999999999645, -12.00000000000000178 ) ) ;
#4520=EDGE_CURVE ( 'NONE', #11190, #12693, #3221, .T. ) ;
#4521=ADVANCED_FACE ( 'NONE', ( #2370 ), #11056, .F. ) ;
#4530=LINE ( 'NONE', #10371, #6250 ) ;
#4533=DIRECTION ( 'NONE',  ( 0.000000000000000000, -1.000000000000000000, 0.000000000000000000 ) ) ;
#4536=AXIS2_PLACEMENT_3D ( 'NONE', #11343, #5660, #3489 ) ;
#4560=EDGE_LOOP ( 'NONE', ( #8725, #2308, #10016, #5358 ) ) ;
#4580=LINE ( 'NONE', #702, #3722 ) ;
#4594=DIRECTION ( 'NONE',  ( 1.000000000000000000, -0.000000000000000000, -6.938893903907228378E-17 ) ) ;
#4600=EDGE_CURVE ( 'NONE', #2451, #1427, #12472, .T. ) ;
#4636=DIRECTION ( 'NONE',  ( 0.000000000000000000, 1.000000000000000000, 0.000000000000000000 ) ) ;
#4640=ORIENTED_EDGE ( 'NONE', *, *, #3203, .F. ) ;
#4642=CARTESIAN_POINT ( 'NONE',  ( 27.00000000000000355, 40.41548023366552655, -10.14535464186970337 ) ) ;
#4646=VECTOR ( 'NONE', #3635, 1000.000000000000000 ) ;
#4661=DIRECTION ( 'NONE',  ( -3.437775699846489820E-17, -0.2951046417778627751, -0.9554649393887560960 ) ) ;
#4677=FACE_OUTER_BOUND ( 'NONE', #4693, .T. ) ;
#4679=EDGE_LOOP ( 'NONE', ( #8303, #2911, #11582, #6243 ) ) ;
#4690=PLANE ( 'NONE',  #6543 ) ;
#4691=DIRECTION ( 'NONE',  ( -2.312964634635743450E-16, 0.9883022714608525883, -0.1525077710325583313 ) ) ;
#4693=EDGE_LOOP ( 'NONE', ( #37, #3162, #3016, #7566 ) ) ;
#4707=ORIENTED_EDGE ( 'NONE', *, *, #8716, .F. ) ;
#4712=LINE ( 'NONE', #2800, #8017 ) ;
#4720=FACE_OUTER_BOUND ( 'NONE', #11764, .T. ) ;
#4730=ORIENTED_EDGE ( 'NONE', *, *, #997, .T. ) ;
#4762=ORIENTED_EDGE ( 'NONE', *, *, #1245, .T. ) ;
#4767=CARTESIAN_POINT ( 'NONE',  ( 33.00000000000000000, 21.47552320888931021, -7.222675303056225182 ) ) ;
#4770=AXIS2_PLACEMENT_3D ( 'NONE', #4133, #7870, #7039 ) ;
#4772=CARTESIAN_POINT ( 'NONE',  ( 40.00000000000000711, 22.56100271565320980, -6.249672610153679919 ) ) ;
#4775=VERTEX_POINT ( 'NONE', #7634 ) ;
#4776=DIRECTION ( 'NONE',  ( 1.000000000000000000, 1.081682119347366197E-16, -6.938893903907228378E-17 ) ) ;
#4792=ORIENTED_EDGE ( 'NONE', *, *, #268, .T. ) ;
#4806=CARTESIAN_POINT ( 'NONE',  ( 27.00000000000000355, 39.34792583643765340, -17.06347054209567560 ) ) ;
#4815=CARTESIAN_POINT ( 'NONE',  ( 40.00000000000000711, 16.67945018363952414, -6.690790236289299919 ) ) ;
#4834=AXIS2_PLACEMENT_3D ( 'NONE', #6113, #10021, #11069 ) ;
#4836=AXIS2_PLACEMENT_3D ( 'NONE', #7068, #6096, #946 ) ;
#4841=FACE_OUTER_BOUND ( 'NONE', #7408, .T. ) ;
#4843=DIRECTION ( 'NONE',  ( -5.208075316782971161E-17, -0.1525077710325583313, -0.9883022714608525883 ) ) ;
#4848=CARTESIAN_POINT ( 'NONE',  ( 20.00000000000000000, 15.24625277455639072, -6.248133273622503481 ) ) ;
#4852=ORIENTED_EDGE ( 'NONE', *, *, #2480, .T. ) ;
#4879=ORIENTED_EDGE ( 'NONE', *, *, #964, .T. ) ;
#4882=CARTESIAN_POINT ( 'NONE',  ( 20.00000000000000355, 14.39651704831740808, -19.59866274153860388 ) ) ;
#4883=AXIS2_PLACEMENT_3D ( 'NONE', #10057, #7880, #2225 ) ;
#4899=CARTESIAN_POINT ( 'NONE',  ( 20.00000000000000355, 21.47552320888931021, -7.222675303056224294 ) ) ;
#4908=VECTOR ( 'NONE', #12347, 1000.000000000000000 ) ;
#4927=FACE_OUTER_BOUND ( 'NONE', #8500, .T. ) ;
#4929=CIRCLE ( 'NONE', #8601, 2.149999999999988809 ) ;
#4933=VERTEX_POINT ( 'NONE', #149 ) ;
#4936=VECTOR ( 'NONE', #9005, 1000.000000000000000 ) ;
#4938=VECTOR ( 'NONE', #2898, 1000.000000000000000 ) ;
#4974=DIRECTION ( 'NONE',  ( 4.703787633549127174E-18, 0.9883022714608525883, -0.1525077710325581370 ) ) ;
#5019=DIRECTION ( 'NONE',  ( 1.000000000000000000, 1.081682119347366321E-16, -6.938893903907228378E-17 ) ) ;
#5024=APPLICATION_CONTEXT ( 'automotive_design' ) ;
#5031=CIRCLE ( 'NONE', #9944, 2.149999999999985256 ) ;
#5068=VERTEX_POINT ( 'NONE', #12397 ) ;
#5084=CARTESIAN_POINT ( 'NONE',  ( 40.00000000000000711, 11.34118543499637255, -24.03007857557328464 ) ) ;
#5097=CARTESIAN_POINT ( 'NONE',  ( 40.00000000000000711, 14.50364731389636574, -24.59751492040896892 ) ) ;
#5100=LINE ( 'NONE', #4130, #11209 ) ;
#5105=ADVANCED_FACE ( 'NONE', ( #12459 ), #7430, .T. ) ;
#5118=CARTESIAN_POINT ( 'NONE',  ( 40.00000000000000711, 15.24625277455639250, -6.248133273622505257 ) ) ;
#5132=DIRECTION ( 'NONE',  ( 0.000000000000000000, 0.000000000000000000, -1.000000000000000000 ) ) ;
#5134=CIRCLE ( 'NONE', #10036, 2.149999999999992362 ) ;
#5154=PRODUCT_DEFINITION_CONTEXT ( 'detailed design', #5918, 'design' ) ;
#5168=CARTESIAN_POINT ( 'NONE',  ( 20.00000000000000000, 15.24625277455639072, -6.248133273622503481 ) ) ;
#5183=EDGE_CURVE ( 'NONE', #8136, #9222, #1984, .T. ) ;
#5200=ORIENTED_EDGE ( 'NONE', *, *, #9825, .F. ) ;
#5202=ORIENTED_EDGE ( 'NONE', *, *, #1472, .T. ) ;
#5204=VERTEX_POINT ( 'NONE', #5743 ) ;
#5208=DIRECTION ( 'NONE',  ( 1.000000000000000000, 1.081682119347366197E-16, -6.938893903907228378E-17 ) ) ;
#5222=DIRECTION ( 'NONE',  ( 0.000000000000000000, 0.000000000000000000, -1.000000000000000000 ) ) ;
#5224=DIRECTION ( 'NONE',  ( 1.238279320584846685E-16, -0.9554649393887558739, 0.2951046417778634412 ) ) ;
#5234=DIRECTION ( 'NONE',  ( -1.238279320584846685E-16, 0.9554649393887558739, -0.2951046417778634412 ) ) ;
#5261=DIRECTION ( 'NONE',  ( 1.238279320584846685E-16, -0.9554649393887560960, 0.2951046417778627751 ) ) ;
#5266=CIRCLE ( 'NONE', #10178, 10.00000000000000178 ) ;
#5271=DIRECTION ( 'NONE',  ( -1.000000000000000000, -1.081682119347366197E-16, 6.938893903907228378E-17 ) ) ;
#5273=CARTESIAN_POINT ( 'NONE',  ( 27.00000000000000355, 39.34792583643766051, -19.21347054209566707 ) ) ;
#5278=ADVANCED_FACE ( 'NONE', ( #5803 ), #15, .F. ) ;
#5300=CARTESIAN_POINT ( 'NONE',  ( 40.00000000000000000, 39.34792583643765340, -17.06347054209567560 ) ) ;
#5302=DIRECTION ( 'NONE',  ( 1.000000000000000000, 1.081682119347366197E-16, -6.938893903907228378E-17 ) ) ;
#5322=VERTEX_POINT ( 'NONE', #6058 ) ;
#5323=DIRECTION ( 'NONE',  ( -1.387778780781445182E-16, 0.9997704357740726522, 0.02142605311579142552 ) ) ;
#5325=EDGE_CURVE ( 'NONE', #1822, #5778, #10819, .T. ) ;
#5326=AXIS2_PLACEMENT_3D ( 'NONE', #1776, #2769, #6808 ) ;
#5332=LINE ( 'NONE', #3297, #10153 ) ;
#5335=EDGE_CURVE ( 'NONE', #11717, #11591, #11018, .T. ) ;
#5338=AXIS2_PLACEMENT_3D ( 'NONE', #10368, #1555, #8445 ) ;
#5353=COLOUR_RGB ( '', 0.31764706, 0.68627451, 0.89019608) ;
#5358=ORIENTED_EDGE ( 'NONE', *, *, #7431, .F. ) ;
#5366=PLANE ( 'NONE',  #12549 ) ;
#5368=CARTESIAN_POINT ( 'NONE',  ( 20.00000000000000000, 9.907988025913237351, -23.58742161290648554 ) ) ;
#5393=ORIENTED_EDGE ( 'NONE', *, *, #6245, .F. ) ;
#5456=ORIENTED_EDGE ( 'NONE', *, *, #12718, .T. ) ;
#5469=UNCERTAINTY_MEASURE_WITH_UNIT (LENGTH_MEASURE( 1.000000000000000082E-05 ), #2406, 'distance_accuracy_value', 'NONE');
#5474=AXIS2_PLACEMENT_3D ( 'NONE', #216, #2289, #6202 ) ;
#5489=EDGE_CURVE ( 'NONE', #11709, #5204, #6314, .T. ) ;
#5496=DIRECTION ( 'NONE',  ( 0.000000000000000000, -1.000000000000000000, 0.000000000000000000 ) ) ;
#5507=VECTOR ( 'NONE', #12620, 1000.000000000000114 ) ;
#5532=ORIENTED_EDGE ( 'NONE', *, *, #10731, .F. ) ;
#5585=FILL_AREA_STYLE ('',( #3599 ) ) ;
#5592=CARTESIAN_POINT ( 'NONE',  ( 27.00000000000000355, 21.47552320888931021, -7.222675303056225182 ) ) ;
#5606=ORIENTED_EDGE ( 'NONE', *, *, #5762, .T. ) ;
#5612=FILL_AREA_STYLE ('',( #3813 ) ) ;
#5616=CARTESIAN_POINT ( 'NONE',  ( 40.00000000000000711, 20.75061298173632451, -7.028257169185711639 ) ) ;
#5622=LINE ( 'NONE', #725, #4103 ) ;
#5623=EDGE_CURVE ( 'NONE', #12693, #5204, #5266, .T. ) ;
#5631=CARTESIAN_POINT ( 'NONE',  ( 40.00000000000000711, 40.41548023366552655, -10.14535464186970692 ) ) ;
#5643=LINE ( 'NONE', #9557, #4938 ) ;
#5645=DIRECTION ( 'NONE',  ( 1.000000000000000000, -0.000000000000000000, -6.938893903907228378E-17 ) ) ;
#5660=DIRECTION ( 'NONE',  ( 1.000000000000000000, 1.081682119347366197E-16, -6.938893903907228378E-17 ) ) ;
#5666=ORIENTED_EDGE ( 'NONE', *, *, #7312, .F. ) ;
#5672=EDGE_CURVE ( 'NONE', #9760, #938, #1462, .T. ) ;
#5685=AXIS2_PLACEMENT_3D ( 'NONE', #2428, #9292, #8590 ) ;
#5690=ADVANCED_FACE ( 'NONE', ( #9307, #2506, #4495 ), #496, .T. ) ;
#5691=DIRECTION ( 'NONE',  ( 0.000000000000000000, 1.000000000000000000, 0.000000000000000000 ) ) ;
#5705=MANIFOLD_SOLID_BREP ( 'M4 Clearance Hole1', #6643 ) ;
#5707=CARTESIAN_POINT ( 'NONE',  ( 0.000000000000000000, 0.000000000000000000, 0.000000000000000000 ) ) ;
#5711=DIRECTION ( 'NONE',  ( -3.437775699846489820E-17, -0.2951046417778627751, -0.9554649393887560960 ) ) ;
#5726=DIRECTION ( 'NONE',  ( 1.000000000000000000, -0.000000000000000000, -6.938893903907228378E-17 ) ) ;
#5731=VERTEX_POINT ( 'NONE', #11054 ) ;
#5736=DIRECTION ( 'NONE',  ( 0.000000000000000000, -0.2951046417778627751, -0.9554649393887560960 ) ) ;
#5743=CARTESIAN_POINT ( 'NONE',  ( 40.00000000000000711, 11.10553687445043103, -10.07215277424222855 ) ) ;
#5753=DIRECTION ( 'NONE',  ( 1.000000000000000000, 1.081682119347366197E-16, -6.938893903907228378E-17 ) ) ;
#5762=EDGE_CURVE ( 'NONE', #6277, #5068, #11654, .T. ) ;
#5763=PLANE ( 'NONE',  #5326 ) ;
#5764=ORIENTED_EDGE ( 'NONE', *, *, #997, .F. ) ;
#5767=ORIENTED_EDGE ( 'NONE', *, *, #3203, .T. ) ;
#5773=LINE ( 'NONE', #11838, #5507 ) ;
#5775=ORIENTED_EDGE ( 'NONE', *, *, #2919, .F. ) ;
#5778=VERTEX_POINT ( 'NONE', #10069 ) ;
#5780=CIRCLE ( 'NONE', #9672, 10.00000000000000178 ) ;
#5791=ORIENTED_EDGE ( 'NONE', *, *, #7038, .F. ) ;
#5801=DIRECTION ( 'NONE',  ( 0.000000000000000000, 0.000000000000000000, -1.000000000000000000 ) ) ;
#5803=FACE_OUTER_BOUND ( 'NONE', #1517, .T. ) ;
#5807=VECTOR ( 'NONE', #10421, 1000.000000000000000 ) ;
#5822=EDGE_CURVE ( 'NONE', #5862, #4933, #11457, .T. ) ;
#5830=ORIENTED_EDGE ( 'NONE', *, *, #6965, .F. ) ;
#5834=ORIENTED_EDGE ( 'NONE', *, *, #5988, .T. ) ;
#5841=CARTESIAN_POINT ( 'NONE',  ( 20.00000000000000355, 20.75061298173632096, -7.028257169185711639 ) ) ;
#5842=CIRCLE ( 'NONE', #8726, 5.000000000000000888 ) ;
#5844=EDGE_LOOP ( 'NONE', ( #103, #12223, #5791, #4120 ) ) ;
#5859=VERTEX_POINT ( 'NONE', #2554 ) ;
#5862=VERTEX_POINT ( 'NONE', #9601 ) ;
#5873=CARTESIAN_POINT ( 'NONE',  ( 27.00000000000000355, 39.34792583643766051, -17.06347054209567915 ) ) ;
#5883=DIRECTION ( 'NONE',  ( 0.000000000000000000, 1.000000000000000000, 0.000000000000000000 ) ) ;
#5914=LINE ( 'NONE', #12632, #8199 ) ;
#5918=APPLICATION_CONTEXT ( 'automotive_design' ) ;
#5934=ADVANCED_FACE ( 'NONE', ( #8526 ), #12470, .F. ) ;
#5937=PRODUCT_DEFINITION ( 'UNKNOWN', '', #7948, #5154 ) ;
#5957=ORIENTED_EDGE ( 'NONE', *, *, #9891, .F. ) ;
#5965=VECTOR ( 'NONE', #2026, 1000.000000000000114 ) ;
#5971=VECTOR ( 'NONE', #1410, 1000.000000000000000 ) ;
#5988=EDGE_CURVE ( 'NONE', #10595, #6024, #6923, .T. ) ;
#5989=CARTESIAN_POINT ( 'NONE',  ( 20.00000000000000000, 8.901672616175321906, -15.56445005073997301 ) ) ;
#5990=CARTESIAN_POINT ( 'NONE',  ( 27.00000000000000355, 30.14235464176399404, -24.26236220746664785 ) ) ;
#6001=DIRECTION ( 'NONE',  ( 2.206481006425900381E-16, -1.000000000000000000, 0.000000000000000000 ) ) ;
#6024=VERTEX_POINT ( 'NONE', #923 ) ;
#6031=VERTEX_POINT ( 'NONE', #8780 ) ;
#6058=CARTESIAN_POINT ( 'NONE',  ( 33.00000000000000000, 30.14235464176399404, -24.26236220746664785 ) ) ;
#6066=VECTOR ( 'NONE', #3609, 1000.000000000000114 ) ;
#6096=DIRECTION ( 'NONE',  ( 1.000000000000000000, 1.081682119347366197E-16, -6.938893903907228378E-17 ) ) ;
#6113=CARTESIAN_POINT ( 'NONE',  ( 40.00000000000000000, 39.34792583643766051, -17.06347054209567915 ) ) ;
#6115=ORIENTED_EDGE ( 'NONE', *, *, #3844, .T. ) ;
#6138=VERTEX_POINT ( 'NONE', #211 ) ;
#6146=ORIENTED_EDGE ( 'NONE', *, *, #3967, .F. ) ;
#6155=CARTESIAN_POINT ( 'NONE',  ( 20.00000000000000355, 10.26855730552413881, -22.42000078613342851 ) ) ;
#6202=DIRECTION ( 'NONE',  ( 0.000000000000000000, -1.000000000000000000, 0.000000000000000000 ) ) ;
#6219=CARTESIAN_POINT ( 'NONE',  ( 20.00000000000000000, 11.34118543499637077, -24.03007857557328464 ) ) ;
#6243=ORIENTED_EDGE ( 'NONE', *, *, #1839, .F. ) ;
#6245=EDGE_CURVE ( 'NONE', #6872, #574, #6463, .T. ) ;
#6250=VECTOR ( 'NONE', #12395, 1000.000000000000000 ) ;
#6254=ORIENTED_EDGE ( 'NONE', *, *, #3842, .F. ) ;
#6265=CARTESIAN_POINT ( 'NONE',  ( 40.00000000000000711, 14.50364731389636574, -24.59751492040896892 ) ) ;
#6268=PRODUCT_DEFINITION_SHAPE ( 'NONE', 'NONE',  #5937 ) ;
#6270=EDGE_LOOP ( 'NONE', ( #3600, #12413, #9238, #2956 ) ) ;
#6277=VERTEX_POINT ( 'NONE', #5616 ) ;
#6282=DIRECTION ( 'NONE',  ( -3.437775699846489820E-17, -0.2951046417778627751, -0.9554649393887560960 ) ) ;
#6289=ORIENTED_EDGE ( 'NONE', *, *, #12183, .F. ) ;
#6307=LINE ( 'NONE', #8243, #7040 ) ;
#6311=AXIS2_PLACEMENT_3D ( 'NONE', #6720, #12588, #11556 ) ;
#6314=LINE ( 'NONE', #1348, #3436 ) ;
#6315=DIRECTION ( 'NONE',  ( -1.000000000000000000, -1.081682119347366197E-16, 6.938893903907228378E-17 ) ) ;
#6360=LINE ( 'NONE', #567, #9628 ) ;
#6379=VECTOR ( 'NONE', #577, 1000.000000000000000 ) ;
#6384=ORIENTED_EDGE ( 'NONE', *, *, #11480, .T. ) ;
#6390=( NAMED_UNIT ( * ) PLANE_ANGLE_UNIT ( ) SI_UNIT ( $, .RADIAN. ) );
#6394=CARTESIAN_POINT ( 'NONE',  ( 40.00000000000000711, 40.41548023366552655, -10.14535464186970692 ) ) ;
#6396=( GEOMETRIC_REPRESENTATION_CONTEXT ( 3 ) GLOBAL_UNCERTAINTY_ASSIGNED_CONTEXT ( ( #6634 ) ) GLOBAL_UNIT_ASSIGNED_CONTEXT ( ( #10560, #8639, #11483 ) ) REPRESENTATION_CONTEXT ( 'NONE', 'WORKASPACE' ) );
#6402=ORIENTED_EDGE ( 'NONE', *, *, #6586, .F. ) ;
#6422=LINE ( 'NONE', #3344, #4113 ) ;
#6428=DIRECTION ( 'NONE',  ( 1.000000000000000000, 0.000000000000000000, 0.000000000000000000 ) ) ;
#6445=PLANE ( 'NONE',  #7666 ) ;
#6463=LINE ( 'NONE', #9279, #563 ) ;
#6476=ORIENTED_EDGE ( 'NONE', *, *, #112, .T. ) ;
#6495=DIRECTION ( 'NONE',  ( 1.000000000000000000, -0.000000000000000000, -6.938893903907228378E-17 ) ) ;
#6509=CARTESIAN_POINT ( 'NONE',  ( 20.00000000000000355, 14.50364731389636397, -24.59751492040896892 ) ) ;
#6543=AXIS2_PLACEMENT_3D ( 'NONE', #8610, #12556, #500 ) ;
#6548=ORIENTED_EDGE ( 'NONE', *, *, #1873, .T. ) ;
#6553=DIRECTION ( 'NONE',  ( -3.437775699846489820E-17, -0.2951046417778627751, -0.9554649393887560960 ) ) ;
#6568=CIRCLE ( 'NONE', #6975, 6.999999999999999112 ) ;
#6584=EDGE_LOOP ( 'NONE', ( #4496, #9536, #5767, #9119 ) ) ;
#6586=EDGE_CURVE ( 'NONE', #12298, #11175, #5332, .T. ) ;
#6608=EDGE_LOOP ( 'NONE', ( #557, #12046, #10932, #4052 ) ) ;
#6619=VERTEX_POINT ( 'NONE', #570 ) ;
#6627=LINE ( 'NONE', #10537, #7185 ) ;
#6630=EDGE_LOOP ( 'NONE', ( #9499, #11510 ) ) ;
#6634=UNCERTAINTY_MEASURE_WITH_UNIT (LENGTH_MEASURE( 1.000000000000000082E-05 ), #10560, 'distance_accuracy_value', 'NONE');
#6638=ORIENTED_EDGE ( 'NONE', *, *, #4317, .F. ) ;
#6642=LINE ( 'NONE', #9447, #6379 ) ;
#6643=CLOSED_SHELL ( 'NONE', ( #8273, #11544, #3922, #8299, #10085, #5105, #948, #220, #7496, #5278, #10403, #367, #7416, #5690, #6864, #12661, #2727, #11484, #10191, #10012, #6915, #2193, #4281, #12268, #11122, #10355, #5934, #10526, #7711, #9846, #3620, #8053, #4521, #615 ) ) ;
#6657=CARTESIAN_POINT ( 'NONE',  ( 33.00000000000000000, 32.50906206197875292, -8.925292473609250266 ) ) ;
#6675=VERTEX_POINT ( 'NONE', #7582 ) ;
#6687=EDGE_CURVE ( 'NONE', #12468, #2451, #9623, .T. ) ;
#6711=CARTESIAN_POINT ( 'NONE',  ( 20.00000000000000000, 10.63631887905125950, -9.927230231572497843 ) ) ;
#6714=SURFACE_STYLE_FILL_AREA ( #5612 ) ;
#6715=DIRECTION ( 'NONE',  ( -3.437775699846489820E-17, -0.2951046417778627751, -0.9554649393887560960 ) ) ;
#6716=PLANE ( 'NONE',  #2938 ) ;
#6720=CARTESIAN_POINT ( 'NONE',  ( 32.99999999999999289, 39.34792583643766051, -17.06347054209567915 ) ) ;
#6738=EDGE_CURVE ( 'NONE', #12468, #2127, #3790, .T. ) ;
#6755=ORIENTED_EDGE ( 'NONE', *, *, #9809, .T. ) ;
#6772=ORIENTED_EDGE ( 'NONE', *, *, #10226, .T. ) ;
#6797=CARTESIAN_POINT ( 'NONE',  ( 20.00000000000000000, 8.901672616175321906, -15.56445005073997301 ) ) ;
#6798=DIRECTION ( 'NONE',  ( 1.000000000000000000, 1.081682119347366197E-16, -6.938893903907228378E-17 ) ) ;
#6808=DIRECTION ( 'NONE',  ( 0.000000000000000000, 0.9554649393887557629, -0.2951046417778634412 ) ) ;
#6823=VERTEX_POINT ( 'NONE', #170 ) ;
#6832=LINE ( 'NONE', #767, #3704 ) ;
#6856=ORIENTED_EDGE ( 'NONE', *, *, #964, .F. ) ;
#6857=VERTEX_POINT ( 'NONE', #5841 ) ;
#6864=ADVANCED_FACE ( 'NONE', ( #6945, #11970, #10791 ), #9880, .F. ) ;
#6869=VECTOR ( 'NONE', #10518, 1000.000000000000000 ) ;
#6872=VERTEX_POINT ( 'NONE', #4095 ) ;
#6880=VECTOR ( 'NONE', #11423, 1000.000000000000114 ) ;
#6897=EDGE_CURVE ( 'NONE', #3836, #12298, #8335, .T. ) ;
#6901=LINE ( 'NONE', #1869, #4936 ) ;
#6915=ADVANCED_FACE ( 'NONE', ( #9115 ), #10132, .F. ) ;
#6923=LINE ( 'NONE', #6797, #553 ) ;
#6945=FACE_BOUND ( 'NONE', #8992, .T. ) ;
#6950=ORIENTED_EDGE ( 'NONE', *, *, #2147, .T. ) ;
#6954=CARTESIAN_POINT ( 'NONE',  ( 20.00000000000000000, 15.24625277455639072, -6.248133273622503481 ) ) ;
#6962=AXIS2_PLACEMENT_3D ( 'NONE', #4163, #1192, #10253 ) ;
#6965=EDGE_CURVE ( 'NONE', #6024, #11591, #4227, .T. ) ;
#6975=AXIS2_PLACEMENT_3D ( 'NONE', #4806, #8730, #7766 ) ;
#6979=VERTEX_POINT ( 'NONE', #1322 ) ;
#6980=CARTESIAN_POINT ( 'NONE',  ( 32.99999999999999289, 44.40501137213340144, -30.19113521482024964 ) ) ;
#6981=CARTESIAN_POINT ( 'NONE',  ( 20.00000000000000355, 18.52447679111067913, -16.77732469694377926 ) ) ;
#7005=VERTEX_POINT ( 'NONE', #6155 ) ;
#7020=ORIENTED_EDGE ( 'NONE', *, *, #6897, .F. ) ;
#7027=ORIENTED_EDGE ( 'NONE', *, *, #4600, .T. ) ;
#7038=EDGE_CURVE ( 'NONE', #9690, #11281, #7325, .T. ) ;
#7039=DIRECTION ( 'NONE',  ( 0.000000000000000000, 0.000000000000000000, -1.000000000000000000 ) ) ;
#7040=VECTOR ( 'NONE', #11273, 1000.000000000000000 ) ;
#7042=ORIENTED_EDGE ( 'NONE', *, *, #4520, .F. ) ;
#7068=CARTESIAN_POINT ( 'NONE',  ( 20.00000000000000355, 18.52447679111067913, -16.77732469694377926 ) ) ;
#7073=ORIENTED_EDGE ( 'NONE', *, *, #5489, .F. ) ;
#7097=DIRECTION ( 'NONE',  ( -1.000000000000000000, -1.081682119347366197E-16, 6.938893903907228378E-17 ) ) ;
#7107=CIRCLE ( 'NONE', #10602, 6.999999999999999112 ) ;
#7108=DIRECTION ( 'NONE',  ( 1.000000000000000000, 1.081682119347366321E-16, -6.938893903907228378E-17 ) ) ;
#7115=DIRECTION ( 'NONE',  ( 1.000000000000000000, 1.081682119347366197E-16, -6.938893903907228378E-17 ) ) ;
#7133=DIRECTION ( 'NONE',  ( -3.437775699846489820E-17, -0.2951046417778627751, -0.9554649393887560960 ) ) ;
#7156=LINE ( 'NONE', #2629, #11081 ) ;
#7162=FACE_OUTER_BOUND ( 'NONE', #6584, .T. ) ;
#7185=VECTOR ( 'NONE', #5711, 1000.000000000000114 ) ;
#7194=CARTESIAN_POINT ( 'NONE',  ( 20.00000000000000000, 22.22477142302764008, -7.338293953734278396 ) ) ;
#7215=DIRECTION ( 'NONE',  ( -1.387778780781445182E-16, 0.9997704357740726522, 0.02142605311579142552 ) ) ;
#7224=LINE ( 'NONE', #12117, #9903 ) ;
#7271=PLANE ( 'NONE',  #8484 ) ;
#7312=EDGE_CURVE ( 'NONE', #6675, #9760, #8195, .T. ) ;
#7316=ORIENTED_EDGE ( 'NONE', *, *, #2550, .T. ) ;
#7319=VERTEX_POINT ( 'NONE', #6265 ) ;
#7325=LINE ( 'NONE', #614, #1138 ) ;
#7330=ORIENTED_EDGE ( 'NONE', *, *, #10773, .F. ) ;
#7333=DIRECTION ( 'NONE',  ( -1.000000000000000000, -1.081682119347366444E-16, 6.938893903907229610E-17 ) ) ;
#7341=CARTESIAN_POINT ( 'NONE',  ( 40.00000000000000711, 8.901672616175323682, -15.56445005073997478 ) ) ;
#7359=AXIS2_PLACEMENT_3D ( 'NONE', #3088, #12096, #5132 ) ;
#7365=LINE ( 'NONE', #3691, #60 ) ;
#7372=ORIENTED_EDGE ( 'NONE', *, *, #3258, .F. ) ;
#7385=VECTOR ( 'NONE', #10404, 1000.000000000000000 ) ;
#7392=DIRECTION ( 'NONE',  ( 0.000000000000000000, 0.000000000000000000, 1.000000000000000000 ) ) ;
#7398=VECTOR ( 'NONE', #3024, 1000.000000000000000 ) ;
#7405=DIRECTION ( 'NONE',  ( -1.000000000000000000, -2.206481006425900381E-16, 8.674603474570138454E-17 ) ) ;
#7408=EDGE_LOOP ( 'NONE', ( #5775, #2899, #9242, #9935, #4425, #12625, #1899, #2504 ) ) ;
#7416=ADVANCED_FACE ( 'NONE', ( #3450 ), #11100, .T. ) ;
#7430=CYLINDRICAL_SURFACE ( 'NONE', #11035, 10.00000000000000000 ) ;
#7431=EDGE_CURVE ( 'NONE', #8682, #6675, #7107, .T. ) ;
#7463=VECTOR ( 'NONE', #7108, 1000.000000000000000 ) ;
#7487=LINE ( 'NONE', #11161, #6880 ) ;
#7496=ADVANCED_FACE ( 'NONE', ( #4720 ), #1563, .T. ) ;
#7497=AXIS2_PLACEMENT_3D ( 'NONE', #7924, #4974, #8713 ) ;
#7520=CARTESIAN_POINT ( 'NONE',  ( 20.00000000000000355, 40.41548023366552655, -10.14535464186970515 ) ) ;
#7542=CARTESIAN_POINT ( 'NONE',  ( 40.00000000000000711, 18.52447679111068268, -16.77732469694377926 ) ) ;
#7557=DIRECTION ( 'NONE',  ( 0.000000000000000000, 0.9554649393887557629, -0.2951046417778634412 ) ) ;
#7560=ORIENTED_EDGE ( 'NONE', *, *, #4351, .T. ) ;
#7566=ORIENTED_EDGE ( 'NONE', *, *, #3967, .T. ) ;
#7574=ORIENTED_EDGE ( 'NONE', *, *, #2637, .F. ) ;
#7582=CARTESIAN_POINT ( 'NONE',  ( 40.00000000000000711, 40.41548023366552655, -10.14535464186970692 ) ) ;
#7584=EDGE_CURVE ( 'NONE', #5731, #6619, #3225, .T. ) ;
#7602=EDGE_CURVE ( 'NONE', #1279, #6823, #8512, .T. ) ;
#7634=CARTESIAN_POINT ( 'NONE',  ( 40.00000000000000711, 8.524480296082934672, -16.78569723734484143 ) ) ;
#7666=AXIS2_PLACEMENT_3D ( 'NONE', #10352, #575, #12500 ) ;
#7696=EDGE_LOOP ( 'NONE', ( #3992, #316, #11782, #7372, #12487, #728, #7706, #5957, #2852, #6384, #6115, #11761, #12105, #10125, #5202, #7330, #8038, #6402, #7020, #9537, #4441, #12616 ) ) ;
#7706=ORIENTED_EDGE ( 'NONE', *, *, #925, .T. ) ;
#7711=ADVANCED_FACE ( 'NONE', ( #3821 ), #2004, .T. ) ;
#7753=PLANE ( 'NONE',  #32 ) ;
#7755=ORIENTED_EDGE ( 'NONE', *, *, #5822, .T. ) ;
#7764=ORIENTED_EDGE ( 'NONE', *, *, #3539, .T. ) ;
#7766=DIRECTION ( 'NONE',  ( 0.000000000000000000, -1.000000000000000000, 0.000000000000000000 ) ) ;
#7769=VECTOR ( 'NONE', #7133, 1000.000000000000114 ) ;
#7814=EDGE_CURVE ( 'NONE', #5068, #5859, #5100, .T. ) ;
#7816=AXIS2_PLACEMENT_3D ( 'NONE', #616, #11444, #12608 ) ;
#7849=ORIENTED_EDGE ( 'NONE', *, *, #895, .T. ) ;
#7870=DIRECTION ( 'NONE',  ( 1.000000000000000000, -0.000000000000000000, -6.938893903907228378E-17 ) ) ;
#7880=DIRECTION ( 'NONE',  ( -1.000000000000000000, -1.081682119347366197E-16, 6.938893903907228378E-17 ) ) ;
#7882=AXIS2_PLACEMENT_3D ( 'NONE', #6980, #2148, #6001 ) ;
#7886=ORIENTED_EDGE ( 'NONE', *, *, #3433, .T. ) ;
#7897=ORIENTED_EDGE ( 'NONE', *, *, #2520, .T. ) ;
#7900=ORIENTED_EDGE ( 'NONE', *, *, #8716, .T. ) ;
#7924=CARTESIAN_POINT ( 'NONE',  ( 33.00000000000000000, 29.58047730022061472, -27.90351864933187898 ) ) ;
#7939=CARTESIAN_POINT ( 'NONE',  ( 40.00000000000000000, 39.34792583643766051, -14.91347054209568945 ) ) ;
#7948=PRODUCT_DEFINITION_FORMATION_WITH_SPECIFIED_SOURCE ( 'ANY', '', #10271, .NOT_KNOWN. ) ;
#8007=ORIENTED_EDGE ( 'NONE', *, *, #5822, .F. ) ;
#8017=VECTOR ( 'NONE', #6715, 1000.000000000000114 ) ;
#8024=AXIS2_PLACEMENT_3D ( 'NONE', #11270, #7405, #3485 ) ;
#8038=ORIENTED_EDGE ( 'NONE', *, *, #12324, .F. ) ;
#8053=ADVANCED_FACE ( 'NONE', ( #8566 ), #580, .F. ) ;
#8060=ORIENTED_EDGE ( 'NONE', *, *, #10919, .T. ) ;
#8066=EDGE_CURVE ( 'NONE', #9690, #11825, #12445, .T. ) ;
#8094=CARTESIAN_POINT ( 'NONE',  ( 40.00000000000000711, 18.52447679111068268, -16.77732469694377926 ) ) ;
#8100=CARTESIAN_POINT ( 'NONE',  ( 40.00000000000000711, 18.52447679111068268, -16.77732469694377926 ) ) ;
#8116=CARTESIAN_POINT ( 'NONE',  ( 20.00000000000000000, 39.34792583643766051, -19.21347054209566707 ) ) ;
#8136=VERTEX_POINT ( 'NONE', #1986 ) ;
#8151=CARTESIAN_POINT ( 'NONE',  ( 20.00000000000000000, 8.163911011730665024, -17.95311239921186441 ) ) ;
#8164=DIRECTION ( 'NONE',  ( 0.000000000000000000, -0.2951046417778627751, -0.9554649393887560960 ) ) ;
#8177=ORIENTED_EDGE ( 'NONE', *, *, #2919, .T. ) ;
#8195=LINE ( 'NONE', #3329, #12261 ) ;
#8199=VECTOR ( 'NONE', #3038, 1000.000000000000000 ) ;
#8203=AXIS2_PLACEMENT_3D ( 'NONE', #12367, #5645, #11583 ) ;
#8243=CARTESIAN_POINT ( 'NONE',  ( 40.00000000000000711, 8.611173066148738897, -18.09125363591105540 ) ) ;
#8273=ADVANCED_FACE ( 'NONE', ( #2190 ), #10147, .F. ) ;
#8281=DIRECTION ( 'NONE',  ( -1.000000000000000000, -2.206481006425900381E-16, 8.674603474570138454E-17 ) ) ;
#8289=( NAMED_UNIT ( * ) SI_UNIT ( $, .STERADIAN. ) SOLID_ANGLE_UNIT ( ) );
#8292=ORIENTED_EDGE ( 'NONE', *, *, #12324, .T. ) ;
#8299=ADVANCED_FACE ( 'NONE', ( #2323 ), #1340, .T. ) ;
#8303=ORIENTED_EDGE ( 'NONE', *, *, #5623, .F. ) ;
#8335=CIRCLE ( 'NONE', #9144, 4.999999999999999112 ) ;
#8347=ORIENTED_EDGE ( 'NONE', *, *, #2637, .T. ) ;
#8348=VERTEX_POINT ( 'NONE', #9436 ) ;
#8357=ORIENTED_EDGE ( 'NONE', *, *, #8745, .F. ) ;
#8371=AXIS2_PLACEMENT_3D ( 'NONE', #9716, #4843, #8826 ) ;
#8400=DIRECTION ( 'NONE',  ( 0.000000000000000000, -0.2951046417778627751, -0.9554649393887560960 ) ) ;
#8411=ORIENTED_EDGE ( 'NONE', *, *, #4317, .T. ) ;
#8415=SURFACE_STYLE_USAGE ( .BOTH. , #433 ) ;
#8429=ORIENTED_EDGE ( 'NONE', *, *, #7602, .F. ) ;
#8439=EDGE_CURVE ( 'NONE', #4775, #11591, #9254, .T. ) ;
#8440=ORIENTED_EDGE ( 'NONE', *, *, #5762, .F. ) ;
#8445=DIRECTION ( 'NONE',  ( 0.000000000000000000, 1.000000000000000000, 0.000000000000000000 ) ) ;
#8451=DIRECTION ( 'NONE',  ( -1.000000000000000000, -1.081682119347366197E-16, 6.938893903907228378E-17 ) ) ;
#8453=EDGE_CURVE ( 'NONE', #8729, #6857, #11462, .T. ) ;
#8474=( NAMED_UNIT ( * ) PLANE_ANGLE_UNIT ( ) SI_UNIT ( $, .RADIAN. ) );
#8484=AXIS2_PLACEMENT_3D ( 'NONE', #12040, #5261, #431 ) ;
#8489=ORIENTED_EDGE ( 'NONE', *, *, #872, .T. ) ;
#8494=DIRECTION ( 'NONE',  ( 5.208075316782974243E-17, 0.1525077710325581370, 0.9883022714608525883 ) ) ;
#8495=AXIS2_PLACEMENT_3D ( 'NONE', #4494, #6495, #9424 ) ;
#8500=EDGE_LOOP ( 'NONE', ( #2854, #6476, #7316, #1714 ) ) ;
#8503=EDGE_CURVE ( 'NONE', #3286, #6138, #10211, .T. ) ;
#8512=LINE ( 'NONE', #12461, #4646 ) ;
#8515=LINE ( 'NONE', #10697, #10880 ) ;
#8522=VECTOR ( 'NONE', #4691, 1000.000000000000000 ) ;
#8526=FACE_OUTER_BOUND ( 'NONE', #6270, .T. ) ;
#8527=LINE ( 'NONE', #3647, #4908 ) ;
#8554=ORIENTED_EDGE ( 'NONE', *, *, #62, .F. ) ;
#8566=FACE_OUTER_BOUND ( 'NONE', #9319, .T. ) ;
#8588=ORIENTED_EDGE ( 'NONE', *, *, #4351, .F. ) ;
#8589=CARTESIAN_POINT ( 'NONE',  ( 40.00000000000000711, 18.52447679111068268, -16.77732469694377926 ) ) ;
#8590=DIRECTION ( 'NONE',  ( 0.000000000000000000, 1.000000000000000000, 0.000000000000000000 ) ) ;
#8601=AXIS2_PLACEMENT_3D ( 'NONE', #9635, #5726, #1737 ) ;
#8610=CARTESIAN_POINT ( 'NONE',  ( 20.00000000000000000, 9.597108420813796670, -18.39576936187866352 ) ) ;
#8623=DIRECTION ( 'NONE',  ( -3.437775699846489820E-17, -0.2951046417778627751, -0.9554649393887560960 ) ) ;
#8639=( NAMED_UNIT ( * ) PLANE_ANGLE_UNIT ( ) SI_UNIT ( $, .RADIAN. ) );
#8643=DIRECTION ( 'NONE',  ( 0.000000000000000000, -0.9997704357740726522, -0.02142605311579142205 ) ) ;
#8650=VECTOR ( 'NONE', #5208, 1000.000000000000000 ) ;
#8665=CARTESIAN_POINT ( 'NONE',  ( 20.00000000000000355, 8.524476791110679130, -16.77732469694377926 ) ) ;
#8680=DIRECTION ( 'NONE',  ( 1.000000000000000000, -1.259148358202862343E-17, -5.075416248775500648E-17 ) ) ;
#8682=VERTEX_POINT ( 'NONE', #2483 ) ;
#8702=AXIS2_PLACEMENT_3D ( 'NONE', #11286, #3568, #11553 ) ;
#8713=DIRECTION ( 'NONE',  ( 0.000000000000000000, 0.1525077710325581370, 0.9883022714608525883 ) ) ;
#8716=EDGE_CURVE ( 'NONE', #9151, #3286, #5031, .T. ) ;
#8725=ORIENTED_EDGE ( 'NONE', *, *, #2439, .T. ) ;
#8726=AXIS2_PLACEMENT_3D ( 'NONE', #3205, #7115, #11036 ) ;
#8729=VERTEX_POINT ( 'NONE', #1499 ) ;
#8730=DIRECTION ( 'NONE',  ( -1.000000000000000000, -2.206481006425900381E-16, 8.674603474570138454E-17 ) ) ;
#8732=VECTOR ( 'NONE', #10496, 1000.000000000000000 ) ;
#8744=ORIENTED_EDGE ( 'NONE', *, *, #5335, .T. ) ;
#8745=EDGE_CURVE ( 'NONE', #11042, #7319, #5842, .T. ) ;
#8780=CARTESIAN_POINT ( 'NONE',  ( 32.99999999999999289, 40.41548023366552655, -10.14535464186970692 ) ) ;
#8782=VECTOR ( 'NONE', #5224, 1000.000000000000000 ) ;
#8804=DIRECTION ( 'NONE',  ( 0.000000000000000000, 1.000000000000000000, 0.000000000000000000 ) ) ;
#8806=ORIENTED_EDGE ( 'NONE', *, *, #2792, .T. ) ;
#8826=DIRECTION ( 'NONE',  ( 0.000000000000000000, 0.9883022714608525883, -0.1525077710325583313 ) ) ;
#8832=AXIS2_PLACEMENT_3D ( 'NONE', #2075, #1101, #9973 ) ;
#8852=ORIENTED_EDGE ( 'NONE', *, *, #578, .F. ) ;
#8867=CARTESIAN_POINT ( 'NONE',  ( 27.00000000000000355, 32.50906206197875292, -8.925292473609250266 ) ) ;
#8896=VECTOR ( 'NONE', #1190, 1000.000000000000000 ) ;
#8903=ORIENTED_EDGE ( 'NONE', *, *, #12265, .T. ) ;
#8907=CYLINDRICAL_SURFACE ( 'NONE', #4883, 6.999999999999999112 ) ;
#8959=( GEOMETRIC_REPRESENTATION_CONTEXT ( 3 ) GLOBAL_UNCERTAINTY_ASSIGNED_CONTEXT ( ( #2873 ) ) GLOBAL_UNIT_ASSIGNED_CONTEXT ( ( #11195, #8474, #8289 ) ) REPRESENTATION_CONTEXT ( 'NONE', 'WORKASPACE' ) );
#8961=LINE ( 'NONE', #10046, #7463 ) ;
#8973=EDGE_LOOP ( 'NONE', ( #8429, #6856, #6146, #6755 ) ) ;
#8992=EDGE_LOOP ( 'NONE', ( #7900, #4730 ) ) ;
#8993=ORIENTED_EDGE ( 'NONE', *, *, #8503, .F. ) ;
#9005=DIRECTION ( 'NONE',  ( -1.000000000000000000, -1.081682119347366197E-16, 6.938893903907228378E-17 ) ) ;
#9019=AXIS2_PLACEMENT_3D ( 'NONE', #5873, #2936, #3822 ) ;
#9033=EDGE_CURVE ( 'NONE', #6138, #9558, #1212, .T. ) ;
#9083=DIRECTION ( 'NONE',  ( -3.437775699846481192E-17, -0.2951046417778634967, -0.9554649393887558739 ) ) ;
#9100=CARTESIAN_POINT ( 'NONE',  ( 40.00000000000000711, 18.52447679111068268, -16.77732469694377926 ) ) ;
#9107=EDGE_LOOP ( 'NONE', ( #8993, #4707, #6772, #11384 ) ) ;
#9115=FACE_OUTER_BOUND ( 'NONE', #5844, .T. ) ;
#9119=ORIENTED_EDGE ( 'NONE', *, *, #1479, .T. ) ;
#9144=AXIS2_PLACEMENT_3D ( 'NONE', #4882, #11900, #8804 ) ;
#9151=VERTEX_POINT ( 'NONE', #8116 ) ;
#9160=ORIENTED_EDGE ( 'NONE', *, *, #12188, .F. ) ;
#9182=CARTESIAN_POINT ( 'NONE',  ( 40.00000000000000711, 14.50364731389636574, -24.59751492040896892 ) ) ;
#9216=DIRECTION ( 'NONE',  ( 0.000000000000000000, 1.000000000000000000, 0.000000000000000000 ) ) ;
#9222=VERTEX_POINT ( 'NONE', #2209 ) ;
#9238=ORIENTED_EDGE ( 'NONE', *, *, #3844, .F. ) ;
#9242=ORIENTED_EDGE ( 'NONE', *, *, #872, .F. ) ;
#9254=LINE ( 'NONE', #7341, #6066 ) ;
#9279=CARTESIAN_POINT ( 'NONE',  ( 27.00000000000000355, 14.50364731389636219, -24.59751492040896892 ) ) ;
#9282=CARTESIAN_POINT ( 'NONE',  ( 20.00000000000000000, 39.34792583643766051, -17.06347054209567915 ) ) ;
#9292=DIRECTION ( 'NONE',  ( 1.000000000000000000, 1.081682119347366197E-16, -6.938893903907228378E-17 ) ) ;
#9307=FACE_BOUND ( 'NONE', #2153, .T. ) ;
#9319=EDGE_LOOP ( 'NONE', ( #6638, #8007, #7886, #7849 ) ) ;
#9343=CARTESIAN_POINT ( 'NONE',  ( 40.00000000000000711, 14.39651704831740986, -19.59866274153860388 ) ) ;
#9363=EDGE_LOOP ( 'NONE', ( #8903, #4420, #1438, #3209 ) ) ;
#9382=VECTOR ( 'NONE', #2003, 1000.000000000000114 ) ;
#9409=CARTESIAN_POINT ( 'NONE',  ( 20.00000000000000000, 39.34792583643766051, -14.91347054209568945 ) ) ;
#9410=CARTESIAN_POINT ( 'NONE',  ( 20.00000000000000000, 16.67945018363952059, -6.690790236289298143 ) ) ;
#9424=DIRECTION ( 'NONE',  ( 0.000000000000000000, 0.000000000000000000, -1.000000000000000000 ) ) ;
#9426=VECTOR ( 'NONE', #8623, 1000.000000000000114 ) ;
#9432=ORIENTED_EDGE ( 'NONE', *, *, #2550, .F. ) ;
#9436=CARTESIAN_POINT ( 'NONE',  ( 20.00000000000000000, 16.67945018363952059, -6.690790236289298143 ) ) ;
#9447=CARTESIAN_POINT ( 'NONE',  ( 40.00000000000000000, 39.49790820824818383, -24.06186359251417883 ) ) ;
#9452=DIRECTION ( 'NONE',  ( 1.000000000000000000, -0.000000000000000000, -6.938893903907228378E-17 ) ) ;
#9456=AXIS2_PLACEMENT_3D ( 'NONE', #4019, #3139, #2951 ) ;
#9466=DIRECTION ( 'NONE',  ( -1.000000000000000000, -1.081682119347366197E-16, 6.938893903907228378E-17 ) ) ;
#9471=VERTEX_POINT ( 'NONE', #4772 ) ;
#9499=ORIENTED_EDGE ( 'NONE', *, *, #12666, .T. ) ;
#9501=EDGE_CURVE ( 'NONE', #3728, #6024, #10212, .T. ) ;
#9519=CARTESIAN_POINT ( 'NONE',  ( 20.00000000000000355, 8.524480291341568261, -16.78569157243880383 ) ) ;
#9536=ORIENTED_EDGE ( 'NONE', *, *, #5183, .T. ) ;
#9537=ORIENTED_EDGE ( 'NONE', *, *, #10288, .T. ) ;
#9553=ORIENTED_EDGE ( 'NONE', *, *, #1195, .F. ) ;
#9557=CARTESIAN_POINT ( 'NONE',  ( 40.00000000000000711, 11.10553687445043280, -10.07215277424223032 ) ) ;
#9558=VERTEX_POINT ( 'NONE', #5273 ) ;
#9568=LINE ( 'NONE', #10486, #5807 ) ;
#9584=SURFACE_STYLE_USAGE ( .BOTH. , #12581 ) ;
#9601=CARTESIAN_POINT ( 'NONE',  ( 20.00000000000000355, 19.99999999999999645, -14.14999999999999325 ) ) ;
#9623=LINE ( 'NONE', #5592, #8522 ) ;
#9628=VECTOR ( 'NONE', #12235, 1000.000000000000000 ) ;
#9629=EDGE_LOOP ( 'NONE', ( #5200, #10671 ) ) ;
#9635=CARTESIAN_POINT ( 'NONE',  ( 40.00000000000000711, 19.99999999999999645, -12.00000000000000178 ) ) ;
#9643=ORIENTED_EDGE ( 'NONE', *, *, #2776, .F. ) ;
#9645=VERTEX_POINT ( 'NONE', #1152 ) ;
#9672=AXIS2_PLACEMENT_3D ( 'NONE', #9100, #12080, #10122 ) ;
#9676=CARTESIAN_POINT ( 'NONE',  ( 20.00000000000000000, 22.56100271565320625, -6.249672610153678143 ) ) ;
#9677=ORIENTED_EDGE ( 'NONE', *, *, #10773, .T. ) ;
#9690=VERTEX_POINT ( 'NONE', #12241 ) ;
#9716=CARTESIAN_POINT ( 'NONE',  ( 40.00000000000000711, 21.47552320888931021, -7.222675303056226070 ) ) ;
#9718=EDGE_CURVE ( 'NONE', #6031, #11780, #10062, .T. ) ;
#9755=VECTOR ( 'NONE', #1258, 1000.000000000000000 ) ;
#9756=EDGE_LOOP ( 'NONE', ( #10729, #5393, #2023, #862 ) ) ;
#9760=VERTEX_POINT ( 'NONE', #1599 ) ;
#9786=CARTESIAN_POINT ( 'NONE',  ( 40.00000000000000711, 18.52447679111068268, -16.77732469694377926 ) ) ;
#9804=ORIENTED_EDGE ( 'NONE', *, *, #5623, .T. ) ;
#9805=PRODUCT_CONTEXT ( 'NONE', #5024, 'mechanical' ) ;
#9809=EDGE_CURVE ( 'NONE', #10658, #6823, #6422, .T. ) ;
#9825=EDGE_CURVE ( 'NONE', #9222, #8136, #11732, .T. ) ;
#9846=ADVANCED_FACE ( 'NONE', ( #489, #4419 ), #2373, .F. ) ;
#9847=FACE_OUTER_BOUND ( 'NONE', #2232, .T. ) ;
#9862=ORIENTED_EDGE ( 'NONE', *, *, #8439, .T. ) ;
#9869=EDGE_LOOP ( 'NONE', ( #3858, #8440, #172, #4762 ) ) ;
#9880=PLANE ( 'NONE',  #4836 ) ;
#9891=EDGE_CURVE ( 'NONE', #5778, #2655, #621, .T. ) ;
#9903=VECTOR ( 'NONE', #2329, 1000.000000000000114 ) ;
#9904=LINE ( 'NONE', #5097, #12594 ) ;
#9935=ORIENTED_EDGE ( 'NONE', *, *, #695, .F. ) ;
#9939=VERTEX_POINT ( 'NONE', #8665 ) ;
#9941=CARTESIAN_POINT ( 'NONE',  ( 40.00000000000000711, 15.24625277455639250, -6.248133273622505257 ) ) ;
#9944=AXIS2_PLACEMENT_3D ( 'NONE', #9282, #5302, #407 ) ;
#9946=ORIENTED_EDGE ( 'NONE', *, *, #11215, .T. ) ;
#9973=DIRECTION ( 'NONE',  ( 0.000000000000000000, -0.2951046417778627751, -0.9554649393887560960 ) ) ;
#9977=ORIENTED_EDGE ( 'NONE', *, *, #7584, .F. ) ;
#10012=ADVANCED_FACE ( 'NONE', ( #4927 ), #3959, .F. ) ;
#10016=ORIENTED_EDGE ( 'NONE', *, *, #268, .F. ) ;
#10021=DIRECTION ( 'NONE',  ( 1.000000000000000000, -0.000000000000000000, -6.938893903907228378E-17 ) ) ;
#10036=AXIS2_PLACEMENT_3D ( 'NONE', #1131, #10656, #11835 ) ;
#10045=ORIENTED_EDGE ( 'NONE', *, *, #695, .T. ) ;
#10046=CARTESIAN_POINT ( 'NONE',  ( 20.00000000000000000, 22.56100271565320625, -6.249672610153678143 ) ) ;
#10057=CARTESIAN_POINT ( 'NONE',  ( 40.00000000000000000, 39.34792583643765340, -17.06347054209567560 ) ) ;
#10062=CIRCLE ( 'NONE', #8024, 6.999999999999999112 ) ;
#10069=CARTESIAN_POINT ( 'NONE',  ( 20.00000000000000355, 14.86906044972263352, -7.469374795321336080 ) ) ;
#10076=ORIENTED_EDGE ( 'NONE', *, *, #10919, .F. ) ;
#10085=ADVANCED_FACE ( 'NONE', ( #4212 ), #8907, .T. ) ;
#10097=DIRECTION ( 'NONE',  ( 1.000000000000000000, -0.000000000000000000, -6.938893903907228378E-17 ) ) ;
#10117=AXIS2_PLACEMENT_3D ( 'NONE', #2181, #3415, #11192 ) ;
#10122=DIRECTION ( 'NONE',  ( 0.000000000000000000, 1.000000000000000000, 0.000000000000000000 ) ) ;
#10125=ORIENTED_EDGE ( 'NONE', *, *, #1195, .T. ) ;
#10132=PLANE ( 'NONE',  #2807 ) ;
#10147=CYLINDRICAL_SURFACE ( 'NONE', #4834, 2.149999999999988809 ) ;
#10153=VECTOR ( 'NONE', #7215, 1000.000000000000227 ) ;
#10161=ORIENTED_EDGE ( 'NONE', *, *, #5325, .T. ) ;
#10178=AXIS2_PLACEMENT_3D ( 'NONE', #8094, #10997, #1202 ) ;
#10191=ADVANCED_FACE ( 'NONE', ( #2420 ), #5366, .T. ) ;
#10202=FACE_OUTER_BOUND ( 'NONE', #1698, .T. ) ;
#10211=LINE ( 'NONE', #7939, #1546 ) ;
#10212=LINE ( 'NONE', #3241, #3500 ) ;
#10217=CARTESIAN_POINT ( 'NONE',  ( 20.00000000000000000, 16.67945018363952059, -6.690790236289298143 ) ) ;
#10223=ORIENTED_EDGE ( 'NONE', *, *, #8503, .T. ) ;
#10226=EDGE_CURVE ( 'NONE', #9151, #9558, #8515, .T. ) ;
#10244=ORIENTED_EDGE ( 'NONE', *, *, #2624, .T. ) ;
#10250=DIRECTION ( 'NONE',  ( 0.000000000000000000, 1.000000000000000000, 0.000000000000000000 ) ) ;
#10253=DIRECTION ( 'NONE',  ( 0.000000000000000000, 1.000000000000000000, 0.000000000000000000 ) ) ;
#10271=PRODUCT ( 'Serrated Eccentric Cam Pawl', 'Serrated Eccentric Cam Pawl', '', ( #9805 ) ) ;
#10276=ORIENTED_EDGE ( 'NONE', *, *, #12307, .T. ) ;
#10288=EDGE_CURVE ( 'NONE', #3836, #9690, #5622, .T. ) ;
#10350=ORIENTED_EDGE ( 'NONE', *, *, #6738, .T. ) ;
#10352=CARTESIAN_POINT ( 'NONE',  ( 20.00000000000000000, 10.63631887905125950, -9.927230231572497843 ) ) ;
#10355=ADVANCED_FACE ( 'NONE', ( #11873 ), #3882, .T. ) ;
#10357=DIRECTION ( 'NONE',  ( 2.187388225841179596E-16, -0.9997704357740726522, -0.02142605311579142552 ) ) ;
#10358=VECTOR ( 'NONE', #5019, 1000.000000000000000 ) ;
#10368=CARTESIAN_POINT ( 'NONE',  ( 20.00000000000000355, 18.52447679111067913, -16.77732469694377926 ) ) ;
#10370=DIRECTION ( 'NONE',  ( 1.000000000000000000, 1.081682119347366321E-16, -6.938893903907228378E-17 ) ) ;
#10371=CARTESIAN_POINT ( 'NONE',  ( 40.00000000000000711, 10.26855730552414059, -22.42000078613342851 ) ) ;
#10383=AXIS2_PLACEMENT_3D ( 'NONE', #12589, #4466, #12332 ) ;
#10403=ADVANCED_FACE ( 'NONE', ( #9847 ), #1037, .T. ) ;
#10404=DIRECTION ( 'NONE',  ( 1.000000000000000000, -0.000000000000000000, -6.938893903907228378E-17 ) ) ;
#10405=AXIS2_PLACEMENT_3D ( 'NONE', #421, #4414, #4224 ) ;
#10421=DIRECTION ( 'NONE',  ( -1.000000000000000000, -1.081682119347366197E-16, 6.938893903907228378E-17 ) ) ;
#10486=CARTESIAN_POINT ( 'NONE',  ( 40.00000000000000711, 8.524476791110680907, -16.77732469694377926 ) ) ;
#10490=LINE ( 'NONE', #1735, #9426 ) ;
#10491=AXIS2_PLACEMENT_3D ( 'NONE', #12290, #12226, #11381 ) ;
#10496=DIRECTION ( 'NONE',  ( 1.000000000000000000, 1.081682119347366321E-16, -6.938893903907228378E-17 ) ) ;
#10503=DIRECTION ( 'NONE',  ( -1.000000000000000000, -1.081682119347366197E-16, 6.938893903907228378E-17 ) ) ;
#10518=DIRECTION ( 'NONE',  ( 1.000000000000000000, -0.000000000000000000, -6.938893903907228378E-17 ) ) ;
#10522=DIRECTION ( 'NONE',  ( -1.000000000000000000, -1.081682119347366197E-16, 6.938893903907228378E-17 ) ) ;
#10526=ADVANCED_FACE ( 'NONE', ( #2401 ), #3498, .F. ) ;
#10537=CARTESIAN_POINT ( 'NONE',  ( 20.00000000000000000, 22.56100271565320625, -6.249672610153678143 ) ) ;
#10560=( LENGTH_UNIT ( ) NAMED_UNIT ( * ) SI_UNIT ( .MILLI., .METRE. ) );
#10579=ORIENTED_EDGE ( 'NONE', *, *, #8745, .T. ) ;
#10586=ORIENTED_EDGE ( 'NONE', *, *, #6738, .F. ) ;
#10595=VERTEX_POINT ( 'NONE', #9519 ) ;
#10602=AXIS2_PLACEMENT_3D ( 'NONE', #5300, #11232, #9216 ) ;
#10603=DIRECTION ( 'NONE',  ( 1.000000000000000000, -0.000000000000000000, -6.938893903907228378E-17 ) ) ;
#10611=MECHANICAL_DESIGN_GEOMETRIC_PRESENTATION_REPRESENTATION('',(#1772),#8959);
#10613=ORIENTED_EDGE ( 'NONE', *, *, #12183, .T. ) ;
#10637=CARTESIAN_POINT ( 'NONE',  ( 20.00000000000000000, 21.12780530657007461, -5.807015647486883481 ) ) ;
#10654=CARTESIAN_POINT ( 'NONE',  ( 20.00000000000000000, 15.24625277455639072, -6.248133273622503481 ) ) ;
#10656=DIRECTION ( 'NONE',  ( 1.000000000000000000, 1.081682119347366197E-16, -6.938893903907228378E-17 ) ) ;
#10658=VERTEX_POINT ( 'NONE', #6711 ) ;
#10668=CIRCLE ( 'NONE', #8203, 2.149999999999985256 ) ;
#10669=ORIENTED_EDGE ( 'NONE', *, *, #9501, .F. ) ;
#10671=ORIENTED_EDGE ( 'NONE', *, *, #5183, .F. ) ;
#10697=CARTESIAN_POINT ( 'NONE',  ( 40.00000000000000000, 39.34792583643766051, -19.21347054209566707 ) ) ;
#10719=ORIENTED_EDGE ( 'NONE', *, *, #3258, .T. ) ;
#10729=ORIENTED_EDGE ( 'NONE', *, *, #2520, .F. ) ;
#10731=EDGE_CURVE ( 'NONE', #12693, #5778, #6901, .T. ) ;
#10747=CIRCLE ( 'NONE', #8495, 2.149999999999985256 ) ;
#10772=DIRECTION ( 'NONE',  ( 1.000000000000000000, -0.000000000000000000, -6.938893903907228378E-17 ) ) ;
#10773=EDGE_CURVE ( 'NONE', #1427, #938, #3871, .T. ) ;
#10790=LINE ( 'NONE', #3028, #1597 ) ;
#10791=FACE_OUTER_BOUND ( 'NONE', #7696, .T. ) ;
#10808=AXIS2_PLACEMENT_3D ( 'NONE', #11262, #1656, #1589 ) ;
#10819=LINE ( 'NONE', #1163, #9382 ) ;
#10825=FACE_OUTER_BOUND ( 'NONE', #1008, .T. ) ;
#10846=ORIENTED_EDGE ( 'NONE', *, *, #6897, .T. ) ;
#10863=DIRECTION ( 'NONE',  ( -2.312964634635743450E-16, 0.9883022714608525883, -0.1525077710325583313 ) ) ;
#10880=VECTOR ( 'NONE', #850, 1000.000000000000000 ) ;
#10919=EDGE_CURVE ( 'NONE', #1807, #6277, #7156, .T. ) ;
#10932=ORIENTED_EDGE ( 'NONE', *, *, #304, .T. ) ;
#10935=AXIS2_PLACEMENT_3D ( 'NONE', #7542, #4776, #12389 ) ;
#10952=CIRCLE ( 'NONE', #11789, 6.999999999999999112 ) ;
#10978=LINE ( 'NONE', #2165, #5965 ) ;
#10997=DIRECTION ( 'NONE',  ( 1.000000000000000000, 1.081682119347366197E-16, -6.938893903907228378E-17 ) ) ;
#11018=LINE ( 'NONE', #135, #8782 ) ;
#11024=CYLINDRICAL_SURFACE ( 'NONE', #4770, 2.149999999999988809 ) ;
#11035=AXIS2_PLACEMENT_3D ( 'NONE', #11490, #9466, #5496 ) ;
#11036=DIRECTION ( 'NONE',  ( 0.000000000000000000, 1.000000000000000000, 0.000000000000000000 ) ) ;
#11037=AXIS2_PLACEMENT_3D ( 'NONE', #9410, #3646, #8400 ) ;
#11042=VERTEX_POINT ( 'NONE', #805 ) ;
#11054=CARTESIAN_POINT ( 'NONE',  ( 40.00000000000000711, 19.99999999999999645, -9.850000000000013856 ) ) ;
#11056=CYLINDRICAL_SURFACE ( 'NONE', #7359, 2.149999999999988809 ) ;
#11059=ORIENTED_EDGE ( 'NONE', *, *, #12265, .F. ) ;
#11069=DIRECTION ( 'NONE',  ( 0.000000000000000000, 0.000000000000000000, -1.000000000000000000 ) ) ;
#11080=CYLINDRICAL_SURFACE ( 'NONE', #264, 2.149999999999988809 ) ;
#11081=VECTOR ( 'NONE', #6553, 1000.000000000000114 ) ;
#11088=CARTESIAN_POINT ( 'NONE',  ( 40.00000000000000711, 10.63631887905126128, -9.927230231572499619 ) ) ;
#11095=CARTESIAN_POINT ( 'NONE',  ( 40.00000000000000711, 21.12780530657007816, -5.807015647486885257 ) ) ;
#11100=CYLINDRICAL_SURFACE ( 'NONE', #5474, 6.999999999999999112 ) ;
#11118=DIRECTION ( 'NONE',  ( -1.000000000000000000, -1.081682119347366197E-16, 6.938893903907228378E-17 ) ) ;
#11122=ADVANCED_FACE ( 'NONE', ( #4677 ), #5763, .F. ) ;
#11131=CARTESIAN_POINT ( 'NONE',  ( 20.00000000000000000, 22.56100271565320625, -6.249672610153678143 ) ) ;
#11132=VERTEX_POINT ( 'NONE', #9676 ) ;
#11135=EDGE_CURVE ( 'NONE', #2451, #6872, #6568, .T. ) ;
#11156=CARTESIAN_POINT ( 'NONE',  ( 32.99999999999999289, 39.49790820824818383, -24.06186359251417883 ) ) ;
#11161=CARTESIAN_POINT ( 'NONE',  ( 20.00000000000000000, 16.67945018363952059, -6.690790236289298143 ) ) ;
#11173=EDGE_LOOP ( 'NONE', ( #10350, #8588, #8489, #7897 ) ) ;
#11175=VERTEX_POINT ( 'NONE', #95 ) ;
#11186=CARTESIAN_POINT ( 'NONE',  ( 32.99999999999999289, 39.34792583643766051, -17.06347054209567915 ) ) ;
#11190=VERTEX_POINT ( 'NONE', #5118 ) ;
#11192=DIRECTION ( 'NONE',  ( 0.000000000000000000, -1.000000000000000000, 0.000000000000000000 ) ) ;
#11195=( LENGTH_UNIT ( ) NAMED_UNIT ( * ) SI_UNIT ( .MILLI., .METRE. ) );
#11205=DIRECTION ( 'NONE',  ( 1.238279320584846685E-16, -0.9554649393887558739, 0.2951046417778634412 ) ) ;
#11209=VECTOR ( 'NONE', #6315, 1000.000000000000000 ) ;
#11215=EDGE_CURVE ( 'NONE', #9645, #4775, #5780, .T. ) ;
#11228=LINE ( 'NONE', #4265, #11588 ) ;
#11232=DIRECTION ( 'NONE',  ( 1.000000000000000000, 1.081682119347366197E-16, -6.938893903907228378E-17 ) ) ;
#11262=CARTESIAN_POINT ( 'NONE',  ( 40.00000000000000711, 18.52447679111068268, -16.77732469694377926 ) ) ;
#11270=CARTESIAN_POINT ( 'NONE',  ( 32.99999999999999289, 39.34792583643765340, -17.06347054209567560 ) ) ;
#11273=DIRECTION ( 'NONE',  ( 1.000000000000000000, 1.081682119347366197E-16, -6.938893903907228378E-17 ) ) ;
#11281=VERTEX_POINT ( 'NONE', #5368 ) ;
#11286=CARTESIAN_POINT ( 'NONE',  ( 40.00000000000000711, 18.52447679111068268, -16.77732469694377926 ) ) ;
#11288=AXIS2_PLACEMENT_3D ( 'NONE', #6981, #6798, #5883 ) ;
#11294=DIRECTION ( 'NONE',  ( 0.000000000000000000, -0.2951046417778627751, -0.9554649393887560960 ) ) ;
#11299=ORIENTED_EDGE ( 'NONE', *, *, #10226, .F. ) ;
#11323=EDGE_LOOP ( 'NONE', ( #2768, #3772, #427, #4640 ) ) ;
#11341=LINE ( 'NONE', #511, #460 ) ;
#11343=CARTESIAN_POINT ( 'NONE',  ( 20.00000000000000355, 18.52447679111067913, -16.77732469694377926 ) ) ;
#11381=DIRECTION ( 'NONE',  ( 2.206481006425900381E-16, -1.000000000000000000, 0.000000000000000000 ) ) ;
#11384=ORIENTED_EDGE ( 'NONE', *, *, #9033, .F. ) ;
#11387=VECTOR ( 'NONE', #5323, 1000.000000000000227 ) ;
#11389=SURFACE_STYLE_FILL_AREA ( #5585 ) ;
#11403=AXIS2_PLACEMENT_3D ( 'NONE', #2673, #4594, #5801 ) ;
#11423=DIRECTION ( 'NONE',  ( -3.437775699846489820E-17, -0.2951046417778627751, -0.9554649393887560960 ) ) ;
#11437=DIRECTION ( 'NONE',  ( 1.000000000000000000, 1.081682119347366197E-16, -6.938893903907228378E-17 ) ) ;
#11444=DIRECTION ( 'NONE',  ( 1.000000000000000000, 1.081682119347366197E-16, -6.938893903907228378E-17 ) ) ;
#11457=CIRCLE ( 'NONE', #5685, 2.149999999999992362 ) ;
#11462=LINE ( 'NONE', #505, #2804 ) ;
#11480=EDGE_CURVE ( 'NONE', #1822, #8348, #12595, .T. ) ;
#11483=( NAMED_UNIT ( * ) SI_UNIT ( $, .STERADIAN. ) SOLID_ANGLE_UNIT ( ) );
#11484=ADVANCED_FACE ( 'NONE', ( #1819 ), #7753, .F. ) ;
#11490=CARTESIAN_POINT ( 'NONE',  ( 40.00000000000000711, 18.52447679111068268, -16.77732469694377926 ) ) ;
#11510=ORIENTED_EDGE ( 'NONE', *, *, #9033, .T. ) ;
#11544=ADVANCED_FACE ( 'NONE', ( #10825 ), #11024, .F. ) ;
#11551=( NAMED_UNIT ( * ) SI_UNIT ( $, .STERADIAN. ) SOLID_ANGLE_UNIT ( ) );
#11553=DIRECTION ( 'NONE',  ( 0.000000000000000000, -1.000000000000000000, 0.000000000000000000 ) ) ;
#11556=DIRECTION ( 'NONE',  ( 0.000000000000000000, -1.000000000000000000, 0.000000000000000000 ) ) ;
#11582=ORIENTED_EDGE ( 'NONE', *, *, #9891, .T. ) ;
#11583=DIRECTION ( 'NONE',  ( 0.000000000000000000, 0.000000000000000000, -1.000000000000000000 ) ) ;
#11588=VECTOR ( 'NONE', #4330, 1000.000000000000000 ) ;
#11591=VERTEX_POINT ( 'NONE', #12002 ) ;
#11654=CIRCLE ( 'NONE', #10405, 10.00000000000000178 ) ;
#11671=DIRECTION ( 'NONE',  ( 1.238279320584846685E-16, -0.9554649393887560960, 0.2951046417778627751 ) ) ;
#11673=CYLINDRICAL_SURFACE ( 'NONE', #11403, 2.149999999999992362 ) ;
#11709=VERTEX_POINT ( 'NONE', #11088 ) ;
#11711=VECTOR ( 'NONE', #3799, 1000.000000000000000 ) ;
#11717=VERTEX_POINT ( 'NONE', #3441 ) ;
#11732=CIRCLE ( 'NONE', #1651, 2.149999999999985256 ) ;
#11761=ORIENTED_EDGE ( 'NONE', *, *, #1245, .F. ) ;
#11764=EDGE_LOOP ( 'NONE', ( #3798, #10846, #8852, #8357 ) ) ;
#11771=VECTOR ( 'NONE', #10357, 1000.000000000000227 ) ;
#11780=VERTEX_POINT ( 'NONE', #11156 ) ;
#11782=ORIENTED_EDGE ( 'NONE', *, *, #5988, .F. ) ;
#11789=AXIS2_PLACEMENT_3D ( 'NONE', #3614, #699, #4636 ) ;
#11812=ORIENTED_EDGE ( 'NONE', *, *, #6965, .T. ) ;
#11825=VERTEX_POINT ( 'NONE', #713 ) ;
#11835=DIRECTION ( 'NONE',  ( 0.000000000000000000, 1.000000000000000000, 0.000000000000000000 ) ) ;
#11838=CARTESIAN_POINT ( 'NONE',  ( 33.00000000000000000, 29.58047730022061472, -27.90351864933187898 ) ) ;
#11861=PLANE ( 'NONE',  #821 ) ;
#11867=EDGE_CURVE ( 'NONE', #1279, #9645, #3947, .T. ) ;
#11873=FACE_OUTER_BOUND ( 'NONE', #3919, .T. ) ;
#11894=CARTESIAN_POINT ( 'NONE',  ( 40.00000000000000711, 9.907988025913239127, -23.58742161290648554 ) ) ;
#11900=DIRECTION ( 'NONE',  ( 1.000000000000000000, 1.081682119347366197E-16, -6.938893903907228378E-17 ) ) ;
#11909=CARTESIAN_POINT ( 'NONE',  ( 40.00000000000000711, 8.524480291341571814, -16.78569157243880738 ) ) ;
#11942=FACE_OUTER_BOUND ( 'NONE', #1235, .T. ) ;
#11968=DIRECTION ( 'NONE',  ( -1.000000000000000000, 1.587729746749930812E-17, 7.204735498949985729E-17 ) ) ;
#11970=FACE_BOUND ( 'NONE', #4075, .T. ) ;
#11995=AXIS2_PLACEMENT_3D ( 'NONE', #4348, #11437, #10250 ) ;
#12002=CARTESIAN_POINT ( 'NONE',  ( 40.00000000000000711, 8.163911011730666800, -17.95311239921186441 ) ) ;
#12033=AXIS2_PLACEMENT_3D ( 'NONE', #4515, #9452, #643 ) ;
#12040=CARTESIAN_POINT ( 'NONE',  ( 20.00000000000000000, 21.12780530657007461, -5.807015647486883481 ) ) ;
#12045=LINE ( 'NONE', #11909, #8650 ) ;
#12046=ORIENTED_EDGE ( 'NONE', *, *, #824, .T. ) ;
#12047=AXIS2_PLACEMENT_3D ( 'NONE', #8100, #5271, #12050 ) ;
#12050=DIRECTION ( 'NONE',  ( 0.000000000000000000, -1.000000000000000000, 0.000000000000000000 ) ) ;
#12080=DIRECTION ( 'NONE',  ( 1.000000000000000000, 1.081682119347366197E-16, -6.938893903907228378E-17 ) ) ;
#12083=EDGE_CURVE ( 'NONE', #2021, #6979, #10747, .T. ) ;
#12096=DIRECTION ( 'NONE',  ( 1.000000000000000000, -0.000000000000000000, -6.938893903907228378E-17 ) ) ;
#12105=ORIENTED_EDGE ( 'NONE', *, *, #8453, .F. ) ;
#12117=CARTESIAN_POINT ( 'NONE',  ( 40.00000000000000711, 16.67945018363952414, -6.690790236289299919 ) ) ;
#12128=DIRECTION ( 'NONE',  ( 0.000000000000000000, 0.9554649393887557629, -0.2951046417778634412 ) ) ;
#12151=EDGE_LOOP ( 'NONE', ( #1254, #8411, #2226, #1715 ) ) ;
#12167=ORIENTED_EDGE ( 'NONE', *, *, #1630, .F. ) ;
#12183=EDGE_CURVE ( 'NONE', #3728, #11717, #6307, .T. ) ;
#12188=EDGE_CURVE ( 'NONE', #4291, #5068, #7224, .T. ) ;
#12217=EDGE_LOOP ( 'NONE', ( #4081, #9946, #9862, #12565, #7764, #6950, #9643, #9432, #10579, #5456, #2700, #12278, #950, #8554, #8060, #5606, #9160, #11059, #2689, #9804, #7073, #4879 ) ) ;
#12221=DIRECTION ( 'NONE',  ( -1.238279320584846685E-16, 0.9554649393887558739, -0.2951046417778634412 ) ) ;
#12223=ORIENTED_EDGE ( 'NONE', *, *, #304, .F. ) ;
#12226=DIRECTION ( 'NONE',  ( -1.000000000000000000, -2.206481006425900381E-16, 8.674603474570137221E-17 ) ) ;
#12235=DIRECTION ( 'NONE',  ( -1.000000000000000000, -1.081682119347366197E-16, 6.938893903907228378E-17 ) ) ;
#12241=CARTESIAN_POINT ( 'NONE',  ( 20.00000000000000000, 11.34118543499637077, -24.03007857557328464 ) ) ;
#12261=VECTOR ( 'NONE', #277, 1000.000000000000114 ) ;
#12265=EDGE_CURVE ( 'NONE', #11190, #4291, #11341, .T. ) ;
#12268=ADVANCED_FACE ( 'NONE', ( #4444 ), #6445, .T. ) ;
#12278=ORIENTED_EDGE ( 'NONE', *, *, #7312, .T. ) ;
#12290=CARTESIAN_POINT ( 'NONE',  ( 27.00000000000000000, 44.40501137213340144, -30.19113521482024964 ) ) ;
#12292=ORIENTED_EDGE ( 'NONE', *, *, #12666, .F. ) ;
#12298=VERTEX_POINT ( 'NONE', #6509 ) ;
#12307=EDGE_CURVE ( 'NONE', #9645, #9939, #9568, .T. ) ;
#12324=EDGE_CURVE ( 'NONE', #11175, #1427, #10952, .T. ) ;
#12332=DIRECTION ( 'NONE',  ( 0.000000000000000000, 0.000000000000000000, -1.000000000000000000 ) ) ;
#12347=DIRECTION ( 'NONE',  ( -1.238279320584846685E-16, 0.9554649393887558739, -0.2951046417778634412 ) ) ;
#12365=PRESENTATION_STYLE_ASSIGNMENT (( #8415 ) ) ;
#12367=CARTESIAN_POINT ( 'NONE',  ( 40.00000000000000000, 39.34792583643766051, -17.06347054209567915 ) ) ;
#12369=VERTEX_POINT ( 'NONE', #762 ) ;
#12374=DIRECTION ( 'NONE',  ( -3.437775699846489820E-17, -0.2951046417778627751, -0.9554649393887560960 ) ) ;
#12389=DIRECTION ( 'NONE',  ( 0.000000000000000000, 1.000000000000000000, 0.000000000000000000 ) ) ;
#12395=DIRECTION ( 'NONE',  ( -1.000000000000000000, -1.081682119347366197E-16, 6.938893903907228378E-17 ) ) ;
#12397=CARTESIAN_POINT ( 'NONE',  ( 40.00000000000000711, 16.59466514679920124, -6.965300083364793338 ) ) ;
#12413=ORIENTED_EDGE ( 'NONE', *, *, #7814, .T. ) ;
#12422=AXIS2_PLACEMENT_3D ( 'NONE', #5707, #7392, #6428 ) ;
#12445=LINE ( 'NONE', #12508, #8732 ) ;
#12455=CYLINDRICAL_SURFACE ( 'NONE', #8702, 10.00000000000000000 ) ;
#12459=FACE_OUTER_BOUND ( 'NONE', #9869, .T. ) ;
#12461=CARTESIAN_POINT ( 'NONE',  ( 40.00000000000000711, 10.25912655421750763, -11.14847175327133577 ) ) ;
#12468=VERTEX_POINT ( 'NONE', #8867 ) ;
#12470=PLANE ( 'NONE',  #11037 ) ;
#12472=LINE ( 'NONE', #5631, #2610 ) ;
#12487=ORIENTED_EDGE ( 'NONE', *, *, #2093, .F. ) ;
#12500=DIRECTION ( 'NONE',  ( 0.000000000000000000, -0.2951046417778627751, -0.9554649393887560960 ) ) ;
#12508=CARTESIAN_POINT ( 'NONE',  ( 20.00000000000000000, 11.34118543499637077, -24.03007857557328464 ) ) ;
#12518=LINE ( 'NONE', #779, #10358 ) ;
#12541=ORIENTED_EDGE ( 'NONE', *, *, #2644, .F. ) ;
#12549=AXIS2_PLACEMENT_3D ( 'NONE', #4403, #3454, #11294 ) ;
#12556=DIRECTION ( 'NONE',  ( 3.437775699846481192E-17, 0.2951046417778634967, 0.9554649393887558739 ) ) ;
#12565=ORIENTED_EDGE ( 'NONE', *, *, #5335, .F. ) ;
#12570=STYLED_ITEM ( 'NONE', ( #2665 ), #2206 ) ;
#12581=SURFACE_SIDE_STYLE ('',( #6714 ) ) ;
#12588=DIRECTION ( 'NONE',  ( -1.000000000000000000, -2.206481006425900381E-16, 8.674603474570138454E-17 ) ) ;
#12589=CARTESIAN_POINT ( 'NONE',  ( 40.00000000000000711, 19.99999999999999645, -12.00000000000000178 ) ) ;
#12594=VECTOR ( 'NONE', #7097, 1000.000000000000000 ) ;
#12595=LINE ( 'NONE', #4848, #3745 ) ;
#12601=CARTESIAN_POINT ( 'NONE',  ( 40.00000000000000711, 19.99999999999999645, -14.14999999999999503 ) ) ;
#12608=DIRECTION ( 'NONE',  ( 0.000000000000000000, 1.000000000000000000, 0.000000000000000000 ) ) ;
#12615=CARTESIAN_POINT ( 'NONE',  ( 40.00000000000000711, 21.12780530657007816, -5.807015647486885257 ) ) ;
#12616=ORIENTED_EDGE ( 'NONE', *, *, #824, .F. ) ;
#12620=DIRECTION ( 'NONE',  ( 5.208075316782974243E-17, 0.1525077710325581370, 0.9883022714608525883 ) ) ;
#12625=ORIENTED_EDGE ( 'NONE', *, *, #12718, .F. ) ;
#12626=EDGE_LOOP ( 'NONE', ( #6289, #4852, #6254, #2732 ) ) ;
#12628=CIRCLE ( 'NONE', #11995, 9.999999999999998224 ) ;
#12632=CARTESIAN_POINT ( 'NONE',  ( 20.00000000000000000, 21.12780530657007461, -5.807015647486883481 ) ) ;
#12634=CIRCLE ( 'NONE', #488, 10.00000000000000178 ) ;
#12640=SHAPE_REPRESENTATION_RELATIONSHIP ( 'NONE' , 'NONE' ,  #1377, #2206 ) ;
#12661=ADVANCED_FACE ( 'NONE', ( #10202 ), #7271, .T. ) ;
#12665=ORIENTED_EDGE ( 'NONE', *, *, #11215, .F. ) ;
#12666=EDGE_CURVE ( 'NONE', #9558, #6138, #671, .T. ) ;
#12684=AXIS2_PLACEMENT_3D ( 'NONE', #9343, #8451, #4533 ) ;
#12688=EDGE_LOOP ( 'NONE', ( #243, #8177, #8292, #4388 ) ) ;
#12693=VERTEX_POINT ( 'NONE', #2246 ) ;
#12694=LINE ( 'NONE', #6954, #11711 ) ;
#12718=EDGE_CURVE ( 'NONE', #7319, #8682, #3288, .T. ) ;
#12731=ORIENTED_EDGE ( 'NONE', *, *, #1536, .T. ) ;
ENDSEC;
END-ISO-10303-21;
